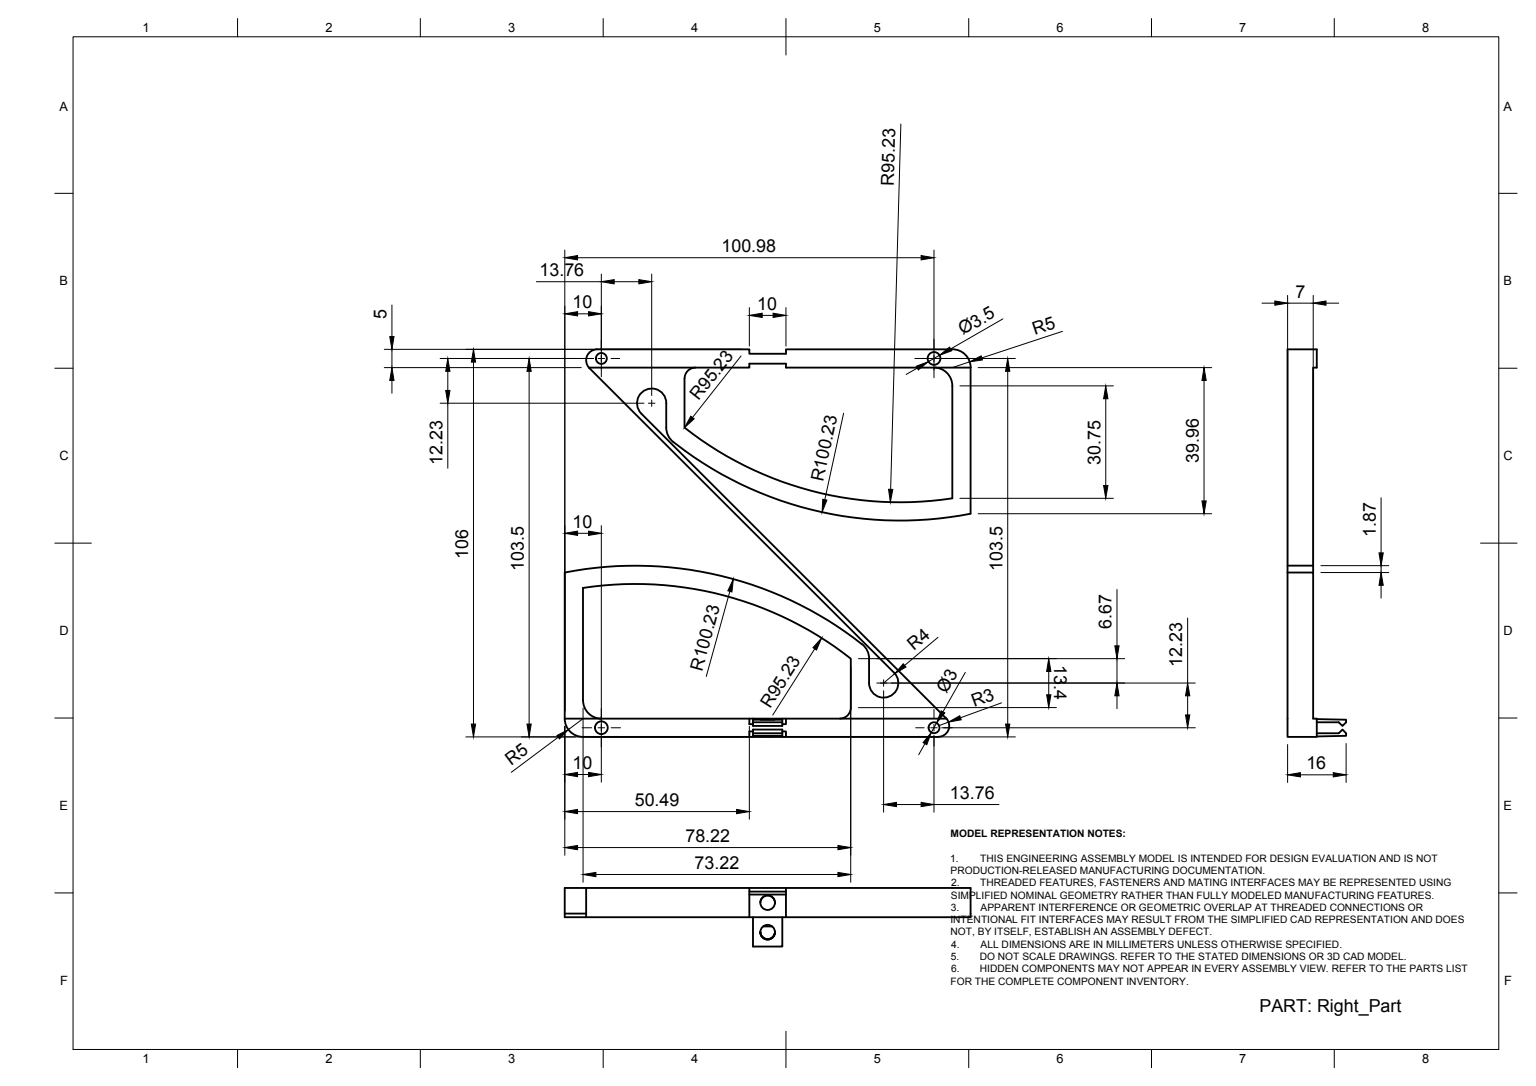
ISO-10303-21;
HEADER;
/* Generated by software containing ST-Developer
 * from STEP Tools, Inc. (www.steptools.com) 
 */

FILE_DESCRIPTION(
/* description */ (''),
/* implementation_level */ '2;1');

FILE_NAME(
/* name */ 'Right_Part.step',
/* time_stamp */ '2026-10-05T13:12:53-07:00',
/* author */ (''),
/* organization */ (''),
/* preprocessor_version */ 'ST-DEVELOPER v20.2',
/* originating_system */ 'Autodesk Translation Framework v15.15.0.0',
/* authorisation */ '');

FILE_SCHEMA (('AUTOMOTIVE_DESIGN { 1 0 10303 214 3 1 1 }'));
ENDSEC;

DATA;
#10=MECHANICAL_DESIGN_GEOMETRIC_PRESENTATION_REPRESENTATION('',(#60),#5912);
#44=SHAPE_REPRESENTATION_RELATIONSHIP('SRR','None',#5945,#52);
#52=ADVANCED_BREP_SHAPE_REPRESENTATION('',(#68),#5905);
#60=STYLED_ITEM('',(#5993),#68);
#68=MANIFOLD_SOLID_BREP('Body1',#3471);
#86=FACE_BOUND('',#473,.T.);
#87=FACE_BOUND('',#474,.T.);
#88=FACE_BOUND('',#485,.T.);
#89=FACE_BOUND('',#489,.T.);
#90=FACE_BOUND('',#510,.T.);
#91=FACE_BOUND('',#511,.T.);
#92=FACE_BOUND('',#513,.T.);
#93=FACE_BOUND('',#515,.T.);
#94=FACE_BOUND('',#516,.T.);
#95=FACE_BOUND('',#522,.T.);
#104=ELLIPSE('',#3708,2.00043399581457,2.);
#105=ELLIPSE('',#3709,2.88922534092348,2.);
#106=ELLIPSE('',#3710,2.00043399581457,2.);
#107=ELLIPSE('',#3711,2.00173692551084,2.);
#108=ELLIPSE('',#3712,2.00173692551084,2.);
#109=ELLIPSE('',#3715,2.00043399581457,2.);
#110=ELLIPSE('',#3716,2.77129645175522,2.);
#111=ELLIPSE('',#3717,2.00043399581457,2.);
#112=ELLIPSE('',#3721,2.00043399581457,2.);
#113=ELLIPSE('',#3722,2.00043399581457,2.);
#138=CYLINDRICAL_SURFACE('',#3707,2.);
#139=CYLINDRICAL_SURFACE('',#3713,2.);
#140=CYLINDRICAL_SURFACE('',#3720,2.);
#141=CYLINDRICAL_SURFACE('',#3723,1.50000013517123);
#142=CYLINDRICAL_SURFACE('',#3727,1.4999996247669);
#143=CYLINDRICAL_SURFACE('',#3732,5.);
#144=CYLINDRICAL_SURFACE('',#3735,5.);
#145=CYLINDRICAL_SURFACE('',#3739,1.75000228959638);
#146=CYLINDRICAL_SURFACE('',#3747,3.00000000000001);
#147=CYLINDRICAL_SURFACE('',#3751,3.99998589024062);
#148=CYLINDRICAL_SURFACE('',#3755,5.00000220964233);
#149=CYLINDRICAL_SURFACE('',#3758,95.231846914414);
#150=CYLINDRICAL_SURFACE('',#3762,3.00000000000008);
#151=CYLINDRICAL_SURFACE('',#3766,2.99999999999999);
#152=CYLINDRICAL_SURFACE('',#3779,100.231846914414);
#153=CYLINDRICAL_SURFACE('',#3794,1.74999969554324);
#154=CYLINDRICAL_SURFACE('',#3798,4.99999999999999);
#155=CYLINDRICAL_SURFACE('',#3801,5.);
#156=CYLINDRICAL_SURFACE('',#3820,100.231846914414);
#157=CYLINDRICAL_SURFACE('',#3832,3.00000000000007);
#158=CYLINDRICAL_SURFACE('',#3834,95.2318469144141);
#159=CYLINDRICAL_SURFACE('',#3836,5.00000220964233);
#160=CYLINDRICAL_SURFACE('',#3838,3.99998589024062);
#161=CYLINDRICAL_SURFACE('',#3840,2.99999999999999);
#250=FACE_OUTER_BOUND('',#443,.T.);
#251=FACE_OUTER_BOUND('',#444,.T.);
#252=FACE_OUTER_BOUND('',#445,.T.);
#253=FACE_OUTER_BOUND('',#446,.T.);
#254=FACE_OUTER_BOUND('',#447,.T.);
#255=FACE_OUTER_BOUND('',#448,.T.);
#256=FACE_OUTER_BOUND('',#449,.T.);
#257=FACE_OUTER_BOUND('',#450,.T.);
#258=FACE_OUTER_BOUND('',#451,.T.);
#259=FACE_OUTER_BOUND('',#452,.T.);
#260=FACE_OUTER_BOUND('',#453,.T.);
#261=FACE_OUTER_BOUND('',#454,.T.);
#262=FACE_OUTER_BOUND('',#455,.T.);
#263=FACE_OUTER_BOUND('',#456,.T.);
#264=FACE_OUTER_BOUND('',#457,.T.);
#265=FACE_OUTER_BOUND('',#458,.T.);
#266=FACE_OUTER_BOUND('',#459,.T.);
#267=FACE_OUTER_BOUND('',#460,.T.);
#268=FACE_OUTER_BOUND('',#461,.T.);
#269=FACE_OUTER_BOUND('',#462,.T.);
#270=FACE_OUTER_BOUND('',#463,.T.);
#271=FACE_OUTER_BOUND('',#464,.T.);
#272=FACE_OUTER_BOUND('',#465,.T.);
#273=FACE_OUTER_BOUND('',#466,.T.);
#274=FACE_OUTER_BOUND('',#467,.T.);
#275=FACE_OUTER_BOUND('',#468,.T.);
#276=FACE_OUTER_BOUND('',#469,.T.);
#277=FACE_OUTER_BOUND('',#470,.T.);
#278=FACE_OUTER_BOUND('',#471,.T.);
#279=FACE_OUTER_BOUND('',#472,.T.);
#280=FACE_OUTER_BOUND('',#475,.T.);
#281=FACE_OUTER_BOUND('',#476,.T.);
#282=FACE_OUTER_BOUND('',#477,.T.);
#283=FACE_OUTER_BOUND('',#478,.T.);
#284=FACE_OUTER_BOUND('',#479,.T.);
#285=FACE_OUTER_BOUND('',#480,.T.);
#286=FACE_OUTER_BOUND('',#481,.T.);
#287=FACE_OUTER_BOUND('',#482,.T.);
#288=FACE_OUTER_BOUND('',#483,.T.);
#289=FACE_OUTER_BOUND('',#484,.T.);
#290=FACE_OUTER_BOUND('',#486,.T.);
#291=FACE_OUTER_BOUND('',#487,.T.);
#292=FACE_OUTER_BOUND('',#488,.T.);
#293=FACE_OUTER_BOUND('',#490,.T.);
#294=FACE_OUTER_BOUND('',#491,.T.);
#295=FACE_OUTER_BOUND('',#492,.T.);
#296=FACE_OUTER_BOUND('',#493,.T.);
#297=FACE_OUTER_BOUND('',#494,.T.);
#298=FACE_OUTER_BOUND('',#495,.T.);
#299=FACE_OUTER_BOUND('',#496,.T.);
#300=FACE_OUTER_BOUND('',#497,.T.);
#301=FACE_OUTER_BOUND('',#498,.T.);
#302=FACE_OUTER_BOUND('',#499,.T.);
#303=FACE_OUTER_BOUND('',#500,.T.);
#304=FACE_OUTER_BOUND('',#501,.T.);
#305=FACE_OUTER_BOUND('',#502,.T.);
#306=FACE_OUTER_BOUND('',#503,.T.);
#307=FACE_OUTER_BOUND('',#504,.T.);
#308=FACE_OUTER_BOUND('',#505,.T.);
#309=FACE_OUTER_BOUND('',#506,.T.);
#310=FACE_OUTER_BOUND('',#507,.T.);
#311=FACE_OUTER_BOUND('',#508,.T.);
#312=FACE_OUTER_BOUND('',#509,.T.);
#313=FACE_OUTER_BOUND('',#512,.T.);
#314=FACE_OUTER_BOUND('',#514,.T.);
#315=FACE_OUTER_BOUND('',#517,.T.);
#316=FACE_OUTER_BOUND('',#518,.T.);
#317=FACE_OUTER_BOUND('',#519,.T.);
#318=FACE_OUTER_BOUND('',#520,.T.);
#319=FACE_OUTER_BOUND('',#521,.T.);
#320=FACE_OUTER_BOUND('',#523,.T.);
#321=FACE_OUTER_BOUND('',#524,.T.);
#322=FACE_OUTER_BOUND('',#525,.T.);
#323=FACE_OUTER_BOUND('',#526,.T.);
#324=FACE_OUTER_BOUND('',#527,.T.);
#325=FACE_OUTER_BOUND('',#528,.T.);
#326=FACE_OUTER_BOUND('',#529,.T.);
#327=FACE_OUTER_BOUND('',#530,.T.);
#328=FACE_OUTER_BOUND('',#531,.T.);
#329=FACE_OUTER_BOUND('',#532,.T.);
#330=FACE_OUTER_BOUND('',#533,.T.);
#331=FACE_OUTER_BOUND('',#534,.T.);
#443=EDGE_LOOP('',(#2654,#2655));
#444=EDGE_LOOP('',(#2656,#2657,#2658,#2659,#2660,#2661,#2662,#2663));
#445=EDGE_LOOP('',(#2664,#2665,#2666,#2667,#2668,#2669));
#446=EDGE_LOOP('',(#2670,#2671,#2672,#2673,#2674,#2675,#2676));
#447=EDGE_LOOP('',(#2677,#2678,#2679,#2680,#2681,#2682,#2683));
#448=EDGE_LOOP('',(#2684,#2685,#2686,#2687));
#449=EDGE_LOOP('',(#2688,#2689,#2690,#2691));
#450=EDGE_LOOP('',(#2692));
#451=EDGE_LOOP('',(#2693,#2694,#2695,#2696));
#452=EDGE_LOOP('',(#2697));
#453=EDGE_LOOP('',(#2698,#2699,#2700,#2701));
#454=EDGE_LOOP('',(#2702,#2703,#2704,#2705,#2706));
#455=EDGE_LOOP('',(#2707,#2708,#2709,#2710));
#456=EDGE_LOOP('',(#2711,#2712,#2713,#2714));
#457=EDGE_LOOP('',(#2715,#2716,#2717,#2718));
#458=EDGE_LOOP('',(#2719));
#459=EDGE_LOOP('',(#2720,#2721,#2722,#2723));
#460=EDGE_LOOP('',(#2724,#2725,#2726,#2727));
#461=EDGE_LOOP('',(#2728,#2729,#2730,#2731,#2732,#2733));
#462=EDGE_LOOP('',(#2734,#2735,#2736,#2737,#2738,#2739));
#463=EDGE_LOOP('',(#2740,#2741,#2742,#2743,#2744));
#464=EDGE_LOOP('',(#2745,#2746,#2747,#2748));
#465=EDGE_LOOP('',(#2749,#2750,#2751,#2752));
#466=EDGE_LOOP('',(#2753,#2754,#2755,#2756));
#467=EDGE_LOOP('',(#2757,#2758,#2759,#2760));
#468=EDGE_LOOP('',(#2761,#2762,#2763,#2764));
#469=EDGE_LOOP('',(#2765,#2766,#2767,#2768));
#470=EDGE_LOOP('',(#2769,#2770,#2771,#2772,#2773,#2774,#2775,#2776,#2777,
#2778,#2779,#2780,#2781,#2782));
#471=EDGE_LOOP('',(#2783,#2784,#2785,#2786));
#472=EDGE_LOOP('',(#2787,#2788,#2789,#2790,#2791,#2792,#2793,#2794,#2795,
#2796,#2797,#2798));
#473=EDGE_LOOP('',(#2799));
#474=EDGE_LOOP('',(#2800));
#475=EDGE_LOOP('',(#2801,#2802,#2803,#2804));
#476=EDGE_LOOP('',(#2805,#2806,#2807,#2808));
#477=EDGE_LOOP('',(#2809,#2810,#2811,#2812));
#478=EDGE_LOOP('',(#2813,#2814,#2815,#2816,#2817,#2818));
#479=EDGE_LOOP('',(#2819,#2820,#2821,#2822,#2823,#2824,#2825,#2826));
#480=EDGE_LOOP('',(#2827,#2828,#2829,#2830,#2831,#2832));
#481=EDGE_LOOP('',(#2833,#2834,#2835,#2836));
#482=EDGE_LOOP('',(#2837,#2838,#2839,#2840));
#483=EDGE_LOOP('',(#2841,#2842,#2843,#2844,#2845,#2846));
#484=EDGE_LOOP('',(#2847,#2848,#2849,#2850));
#485=EDGE_LOOP('',(#2851));
#486=EDGE_LOOP('',(#2852,#2853,#2854,#2855));
#487=EDGE_LOOP('',(#2856,#2857,#2858,#2859,#2860,#2861,#2862,#2863,#2864,
#2865,#2866));
#488=EDGE_LOOP('',(#2867,#2868,#2869,#2870));
#489=EDGE_LOOP('',(#2871,#2872,#2873));
#490=EDGE_LOOP('',(#2874,#2875,#2876,#2877));
#491=EDGE_LOOP('',(#2878,#2879,#2880,#2881));
#492=EDGE_LOOP('',(#2882,#2883,#2884,#2885,#2886,#2887));
#493=EDGE_LOOP('',(#2888,#2889,#2890,#2891,#2892,#2893,#2894,#2895));
#494=EDGE_LOOP('',(#2896,#2897,#2898,#2899));
#495=EDGE_LOOP('',(#2900,#2901,#2902,#2903,#2904,#2905));
#496=EDGE_LOOP('',(#2906,#2907,#2908,#2909,#2910,#2911));
#497=EDGE_LOOP('',(#2912,#2913,#2914,#2915,#2916));
#498=EDGE_LOOP('',(#2917));
#499=EDGE_LOOP('',(#2918,#2919,#2920,#2921));
#500=EDGE_LOOP('',(#2922,#2923,#2924,#2925,#2926,#2927));
#501=EDGE_LOOP('',(#2928,#2929,#2930,#2931));
#502=EDGE_LOOP('',(#2932,#2933,#2934,#2935));
#503=EDGE_LOOP('',(#2936,#2937,#2938,#2939,#2940,#2941));
#504=EDGE_LOOP('',(#2942,#2943,#2944,#2945));
#505=EDGE_LOOP('',(#2946,#2947,#2948,#2949));
#506=EDGE_LOOP('',(#2950,#2951,#2952,#2953));
#507=EDGE_LOOP('',(#2954,#2955,#2956,#2957));
#508=EDGE_LOOP('',(#2958,#2959,#2960,#2961));
#509=EDGE_LOOP('',(#2962,#2963,#2964,#2965,#2966,#2967,#2968,#2969,#2970,
#2971,#2972,#2973,#2974,#2975,#2976,#2977,#2978,#2979,#2980,#2981,#2982,
#2983,#2984));
#510=EDGE_LOOP('',(#2985,#2986,#2987,#2988,#2989,#2990,#2991,#2992,#2993,
#2994));
#511=EDGE_LOOP('',(#2995,#2996,#2997,#2998,#2999,#3000));
#512=EDGE_LOOP('',(#3001,#3002,#3003,#3004));
#513=EDGE_LOOP('',(#3005));
#514=EDGE_LOOP('',(#3006,#3007,#3008,#3009,#3010,#3011,#3012,#3013,#3014,
#3015,#3016,#3017));
#515=EDGE_LOOP('',(#3018));
#516=EDGE_LOOP('',(#3019));
#517=EDGE_LOOP('',(#3020,#3021,#3022,#3023));
#518=EDGE_LOOP('',(#3024,#3025,#3026,#3027));
#519=EDGE_LOOP('',(#3028,#3029,#3030,#3031,#3032,#3033,#3034,#3035,#3036,
#3037,#3038,#3039,#3040,#3041,#3042,#3043,#3044,#3045,#3046,#3047,#3048,
#3049,#3050,#3051,#3052,#3053,#3054,#3055,#3056));
#520=EDGE_LOOP('',(#3057,#3058,#3059,#3060,#3061,#3062));
#521=EDGE_LOOP('',(#3063,#3064,#3065,#3066));
#522=EDGE_LOOP('',(#3067));
#523=EDGE_LOOP('',(#3068,#3069,#3070,#3071,#3072,#3073));
#524=EDGE_LOOP('',(#3074,#3075,#3076,#3077,#3078,#3079));
#525=EDGE_LOOP('',(#3080,#3081,#3082,#3083));
#526=EDGE_LOOP('',(#3084,#3085,#3086,#3087));
#527=EDGE_LOOP('',(#3088,#3089,#3090,#3091));
#528=EDGE_LOOP('',(#3092,#3093,#3094,#3095));
#529=EDGE_LOOP('',(#3096,#3097,#3098,#3099));
#530=EDGE_LOOP('',(#3100,#3101,#3102,#3103));
#531=EDGE_LOOP('',(#3104,#3105,#3106,#3107));
#532=EDGE_LOOP('',(#3108,#3109,#3110,#3111,#3112));
#533=EDGE_LOOP('',(#3113,#3114,#3115,#3116,#3117,#3118,#3119));
#534=EDGE_LOOP('',(#3120,#3121,#3122,#3123));
#598=CIRCLE('',#3706,2.);
#599=CIRCLE('',#3714,2.);
#600=CIRCLE('',#3724,1.50000013517123);
#601=CIRCLE('',#3725,1.50000013517123);
#602=CIRCLE('',#3728,1.4999996247669);
#603=CIRCLE('',#3729,1.4999996247669);
#604=CIRCLE('',#3733,5.);
#605=CIRCLE('',#3734,5.);
#606=CIRCLE('',#3736,5.);
#607=CIRCLE('',#3737,5.);
#608=CIRCLE('',#3740,1.75000228959638);
#609=CIRCLE('',#3741,1.75000228959638);
#610=CIRCLE('',#3748,3.00000000000001);
#611=CIRCLE('',#3749,3.00000000000001);
#612=CIRCLE('',#3750,3.00000000000001);
#613=CIRCLE('',#3752,3.99998589024062);
#614=CIRCLE('',#3753,3.99998589024062);
#615=CIRCLE('',#3756,5.00000220964233);
#616=CIRCLE('',#3757,5.00000220964233);
#617=CIRCLE('',#3759,95.231846914414);
#618=CIRCLE('',#3760,95.231846914414);
#619=CIRCLE('',#3763,3.00000000000008);
#620=CIRCLE('',#3764,3.00000000000008);
#621=CIRCLE('',#3767,2.99999999999999);
#622=CIRCLE('',#3780,100.231846914414);
#623=CIRCLE('',#3781,100.231846914414);
#624=CIRCLE('',#3793,1.74999969554324);
#625=CIRCLE('',#3795,1.74999969554324);
#626=CIRCLE('',#3799,4.99999999999999);
#627=CIRCLE('',#3800,4.99999999999999);
#628=CIRCLE('',#3802,5.);
#629=CIRCLE('',#3803,5.);
#630=CIRCLE('',#3810,2.99999999999999);
#631=CIRCLE('',#3811,100.231846914414);
#632=CIRCLE('',#3812,5.00000220964233);
#633=CIRCLE('',#3813,3.99998589024062);
#634=CIRCLE('',#3814,3.00000000000007);
#635=CIRCLE('',#3815,95.2318469144141);
#636=CIRCLE('',#3818,2.99999999999999);
#637=CIRCLE('',#3821,100.231846914414);
#638=CIRCLE('',#3823,3.99998589024062);
#639=CIRCLE('',#3824,5.00000220964233);
#640=CIRCLE('',#3825,95.2318469144141);
#641=CIRCLE('',#3826,3.00000000000007);
#642=CIRCLE('',#3827,2.99999999999999);
#834=LINE('',#5362,#1199);
#835=LINE('',#5372,#1200);
#836=LINE('',#5379,#1201);
#837=LINE('',#5387,#1202);
#838=LINE('',#5389,#1203);
#839=LINE('',#5391,#1204);
#840=LINE('',#5393,#1205);
#841=LINE('',#5394,#1206);
#842=LINE('',#5397,#1207);
#843=LINE('',#5399,#1208);
#844=LINE('',#5401,#1209);
#845=LINE('',#5403,#1210);
#846=LINE('',#5404,#1211);
#847=LINE('',#5409,#1212);
#848=LINE('',#5415,#1213);
#849=LINE('',#5422,#1214);
#850=LINE('',#5428,#1215);
#851=LINE('',#5430,#1216);
#852=LINE('',#5432,#1217);
#853=LINE('',#5433,#1218);
#854=LINE('',#5438,#1219);
#855=LINE('',#5441,#1220);
#856=LINE('',#5447,#1221);
#857=LINE('',#5450,#1222);
#858=LINE('',#5453,#1223);
#859=LINE('',#5455,#1224);
#860=LINE('',#5456,#1225);
#861=LINE('',#5461,#1226);
#862=LINE('',#5467,#1227);
#863=LINE('',#5469,#1228);
#864=LINE('',#5471,#1229);
#865=LINE('',#5472,#1230);
#866=LINE('',#5476,#1231);
#867=LINE('',#5478,#1232);
#868=LINE('',#5480,#1233);
#869=LINE('',#5481,#1234);
#870=LINE('',#5485,#1235);
#871=LINE('',#5487,#1236);
#872=LINE('',#5488,#1237);
#873=LINE('',#5490,#1238);
#874=LINE('',#5491,#1239);
#875=LINE('',#5495,#1240);
#876=LINE('',#5497,#1241);
#877=LINE('',#5498,#1242);
#878=LINE('',#5500,#1243);
#879=LINE('',#5501,#1244);
#880=LINE('',#5507,#1245);
#881=LINE('',#5512,#1246);
#882=LINE('',#5518,#1247);
#883=LINE('',#5521,#1248);
#884=LINE('',#5524,#1249);
#885=LINE('',#5526,#1250);
#886=LINE('',#5527,#1251);
#887=LINE('',#5532,#1252);
#888=LINE('',#5538,#1253);
#889=LINE('',#5542,#1254);
#890=LINE('',#5544,#1255);
#891=LINE('',#5545,#1256);
#892=LINE('',#5550,#1257);
#893=LINE('',#5554,#1258);
#894=LINE('',#5556,#1259);
#895=LINE('',#5558,#1260);
#896=LINE('',#5560,#1261);
#897=LINE('',#5561,#1262);
#898=LINE('',#5562,#1263);
#899=LINE('',#5563,#1264);
#900=LINE('',#5564,#1265);
#901=LINE('',#5565,#1266);
#902=LINE('',#5566,#1267);
#903=LINE('',#5570,#1268);
#904=LINE('',#5573,#1269);
#905=LINE('',#5575,#1270);
#906=LINE('',#5576,#1271);
#907=LINE('',#5578,#1272);
#908=LINE('',#5579,#1273);
#909=LINE('',#5580,#1274);
#910=LINE('',#5583,#1275);
#911=LINE('',#5584,#1276);
#912=LINE('',#5586,#1277);
#913=LINE('',#5589,#1278);
#914=LINE('',#5591,#1279);
#915=LINE('',#5592,#1280);
#916=LINE('',#5596,#1281);
#917=LINE('',#5598,#1282);
#918=LINE('',#5599,#1283);
#919=LINE('',#5601,#1284);
#920=LINE('',#5602,#1285);
#921=LINE('',#5604,#1286);
#922=LINE('',#5608,#1287);
#923=LINE('',#5610,#1288);
#924=LINE('',#5611,#1289);
#925=LINE('',#5612,#1290);
#926=LINE('',#5614,#1291);
#927=LINE('',#5615,#1292);
#928=LINE('',#5617,#1293);
#929=LINE('',#5624,#1294);
#930=LINE('',#5625,#1295);
#931=LINE('',#5626,#1296);
#932=LINE('',#5627,#1297);
#933=LINE('',#5629,#1298);
#934=LINE('',#5631,#1299);
#935=LINE('',#5633,#1300);
#936=LINE('',#5636,#1301);
#937=LINE('',#5641,#1302);
#938=LINE('',#5643,#1303);
#939=LINE('',#5645,#1304);
#940=LINE('',#5647,#1305);
#941=LINE('',#5649,#1306);
#942=LINE('',#5650,#1307);
#943=LINE('',#5654,#1308);
#944=LINE('',#5656,#1309);
#945=LINE('',#5658,#1310);
#946=LINE('',#5660,#1311);
#947=LINE('',#5662,#1312);
#948=LINE('',#5663,#1313);
#949=LINE('',#5666,#1314);
#950=LINE('',#5668,#1315);
#951=LINE('',#5670,#1316);
#952=LINE('',#5671,#1317);
#953=LINE('',#5677,#1318);
#954=LINE('',#5681,#1319);
#955=LINE('',#5683,#1320);
#956=LINE('',#5685,#1321);
#957=LINE('',#5687,#1322);
#958=LINE('',#5688,#1323);
#959=LINE('',#5692,#1324);
#960=LINE('',#5694,#1325);
#961=LINE('',#5696,#1326);
#962=LINE('',#5697,#1327);
#963=LINE('',#5705,#1328);
#964=LINE('',#5708,#1329);
#965=LINE('',#5710,#1330);
#966=LINE('',#5711,#1331);
#967=LINE('',#5714,#1332);
#968=LINE('',#5716,#1333);
#969=LINE('',#5717,#1334);
#970=LINE('',#5720,#1335);
#971=LINE('',#5721,#1336);
#972=LINE('',#5724,#1337);
#973=LINE('',#5726,#1338);
#974=LINE('',#5727,#1339);
#975=LINE('',#5730,#1340);
#976=LINE('',#5731,#1341);
#977=LINE('',#5734,#1342);
#978=LINE('',#5738,#1343);
#979=LINE('',#5739,#1344);
#980=LINE('',#5743,#1345);
#981=LINE('',#5747,#1346);
#982=LINE('',#5750,#1347);
#983=LINE('',#5752,#1348);
#984=LINE('',#5754,#1349);
#985=LINE('',#5758,#1350);
#986=LINE('',#5762,#1351);
#987=LINE('',#5763,#1352);
#988=LINE('',#5766,#1353);
#989=LINE('',#5768,#1354);
#990=LINE('',#5770,#1355);
#991=LINE('',#5774,#1356);
#992=LINE('',#5775,#1357);
#993=LINE('',#5778,#1358);
#994=LINE('',#5779,#1359);
#995=LINE('',#5783,#1360);
#996=LINE('',#5786,#1361);
#997=LINE('',#5790,#1362);
#998=LINE('',#5793,#1363);
#999=LINE('',#5797,#1364);
#1000=LINE('',#5801,#1365);
#1001=LINE('',#5804,#1366);
#1002=LINE('',#5806,#1367);
#1003=LINE('',#5808,#1368);
#1004=LINE('',#5810,#1369);
#1005=LINE('',#5811,#1370);
#1006=LINE('',#5813,#1371);
#1007=LINE('',#5815,#1372);
#1008=LINE('',#5818,#1373);
#1009=LINE('',#5820,#1374);
#1010=LINE('',#5822,#1375);
#1011=LINE('',#5824,#1376);
#1012=LINE('',#5827,#1377);
#1013=LINE('',#5828,#1378);
#1199=VECTOR('',#4343,10.);
#1200=VECTOR('',#4354,2.);
#1201=VECTOR('',#4363,2.);
#1202=VECTOR('',#4372,10.);
#1203=VECTOR('',#4373,10.);
#1204=VECTOR('',#4374,10.);
#1205=VECTOR('',#4375,10.);
#1206=VECTOR('',#4376,10.);
#1207=VECTOR('',#4379,10.);
#1208=VECTOR('',#4380,10.);
#1209=VECTOR('',#4381,10.);
#1210=VECTOR('',#4382,10.);
#1211=VECTOR('',#4383,10.);
#1212=VECTOR('',#4388,2.);
#1213=VECTOR('',#4395,1.50000013517123);
#1214=VECTOR('',#4404,1.4999996247669);
#1215=VECTOR('',#4411,10.);
#1216=VECTOR('',#4412,10.);
#1217=VECTOR('',#4413,10.);
#1218=VECTOR('',#4414,10.);
#1219=VECTOR('',#4419,10.);
#1220=VECTOR('',#4422,10.);
#1221=VECTOR('',#4427,10.);
#1222=VECTOR('',#4430,10.);
#1223=VECTOR('',#4433,10.);
#1224=VECTOR('',#4434,10.);
#1225=VECTOR('',#4435,10.);
#1226=VECTOR('',#4440,1.75000228959638);
#1227=VECTOR('',#4447,10.);
#1228=VECTOR('',#4448,10.);
#1229=VECTOR('',#4449,10.);
#1230=VECTOR('',#4450,10.);
#1231=VECTOR('',#4453,10.);
#1232=VECTOR('',#4454,10.);
#1233=VECTOR('',#4455,10.);
#1234=VECTOR('',#4456,10.);
#1235=VECTOR('',#4459,10.);
#1236=VECTOR('',#4460,10.);
#1237=VECTOR('',#4461,10.);
#1238=VECTOR('',#4462,10.);
#1239=VECTOR('',#4463,10.);
#1240=VECTOR('',#4466,10.);
#1241=VECTOR('',#4467,10.);
#1242=VECTOR('',#4468,10.);
#1243=VECTOR('',#4469,10.);
#1244=VECTOR('',#4470,10.);
#1245=VECTOR('',#4475,10.);
#1246=VECTOR('',#4480,10.);
#1247=VECTOR('',#4485,10.);
#1248=VECTOR('',#4488,10.);
#1249=VECTOR('',#4491,10.);
#1250=VECTOR('',#4492,10.);
#1251=VECTOR('',#4493,10.);
#1252=VECTOR('',#4498,10.);
#1253=VECTOR('',#4505,10.);
#1254=VECTOR('',#4510,9.99999999999999);
#1255=VECTOR('',#4511,10.);
#1256=VECTOR('',#4512,9.99999999999999);
#1257=VECTOR('',#4517,10.);
#1258=VECTOR('',#4522,10.);
#1259=VECTOR('',#4523,10.);
#1260=VECTOR('',#4524,10.);
#1261=VECTOR('',#4525,10.);
#1262=VECTOR('',#4526,10.);
#1263=VECTOR('',#4527,10.);
#1264=VECTOR('',#4528,10.);
#1265=VECTOR('',#4529,10.);
#1266=VECTOR('',#4530,10.);
#1267=VECTOR('',#4531,10.);
#1268=VECTOR('',#4536,10.);
#1269=VECTOR('',#4539,10.);
#1270=VECTOR('',#4540,10.);
#1271=VECTOR('',#4541,10.);
#1272=VECTOR('',#4542,10.);
#1273=VECTOR('',#4543,10.);
#1274=VECTOR('',#4544,10.);
#1275=VECTOR('',#4547,10.);
#1276=VECTOR('',#4548,10.);
#1277=VECTOR('',#4551,10.);
#1278=VECTOR('',#4554,10.);
#1279=VECTOR('',#4555,10.);
#1280=VECTOR('',#4556,10.);
#1281=VECTOR('',#4559,10.);
#1282=VECTOR('',#4560,10.);
#1283=VECTOR('',#4561,10.);
#1284=VECTOR('',#4562,10.);
#1285=VECTOR('',#4563,10.);
#1286=VECTOR('',#4566,10.);
#1287=VECTOR('',#4569,10.);
#1288=VECTOR('',#4570,10.);
#1289=VECTOR('',#4571,10.);
#1290=VECTOR('',#4572,10.);
#1291=VECTOR('',#4575,10.);
#1292=VECTOR('',#4576,10.);
#1293=VECTOR('',#4579,10.);
#1294=VECTOR('',#4592,10.);
#1295=VECTOR('',#4593,10.);
#1296=VECTOR('',#4594,10.);
#1297=VECTOR('',#4595,10.);
#1298=VECTOR('',#4598,10.);
#1299=VECTOR('',#4601,10.);
#1300=VECTOR('',#4604,10.);
#1301=VECTOR('',#4609,10.);
#1302=VECTOR('',#4614,10.);
#1303=VECTOR('',#4615,10.);
#1304=VECTOR('',#4616,10.);
#1305=VECTOR('',#4617,10.);
#1306=VECTOR('',#4618,10.);
#1307=VECTOR('',#4619,10.);
#1308=VECTOR('',#4622,10.);
#1309=VECTOR('',#4623,10.);
#1310=VECTOR('',#4624,10.);
#1311=VECTOR('',#4625,10.);
#1312=VECTOR('',#4626,10.);
#1313=VECTOR('',#4627,10.);
#1314=VECTOR('',#4630,10.);
#1315=VECTOR('',#4631,10.);
#1316=VECTOR('',#4632,10.);
#1317=VECTOR('',#4633,10.);
#1318=VECTOR('',#4640,1.74999969554324);
#1319=VECTOR('',#4645,10.);
#1320=VECTOR('',#4646,10.);
#1321=VECTOR('',#4647,10.);
#1322=VECTOR('',#4648,10.);
#1323=VECTOR('',#4649,10.);
#1324=VECTOR('',#4652,10.);
#1325=VECTOR('',#4653,10.);
#1326=VECTOR('',#4654,10.);
#1327=VECTOR('',#4655,10.);
#1328=VECTOR('',#4668,10.);
#1329=VECTOR('',#4671,10.);
#1330=VECTOR('',#4672,10.);
#1331=VECTOR('',#4673,10.);
#1332=VECTOR('',#4676,10.);
#1333=VECTOR('',#4677,10.);
#1334=VECTOR('',#4678,10.);
#1335=VECTOR('',#4681,10.);
#1336=VECTOR('',#4682,10.);
#1337=VECTOR('',#4685,10.);
#1338=VECTOR('',#4686,10.);
#1339=VECTOR('',#4687,10.);
#1340=VECTOR('',#4690,10.);
#1341=VECTOR('',#4691,10.);
#1342=VECTOR('',#4694,10.);
#1343=VECTOR('',#4697,10.);
#1344=VECTOR('',#4698,10.);
#1345=VECTOR('',#4701,10.);
#1346=VECTOR('',#4704,10.);
#1347=VECTOR('',#4707,10.);
#1348=VECTOR('',#4708,10.);
#1349=VECTOR('',#4709,10.);
#1350=VECTOR('',#4712,9.99999999999999);
#1351=VECTOR('',#4717,10.);
#1352=VECTOR('',#4718,10.);
#1353=VECTOR('',#4721,10.);
#1354=VECTOR('',#4722,10.);
#1355=VECTOR('',#4723,10.);
#1356=VECTOR('',#4726,10.);
#1357=VECTOR('',#4727,10.);
#1358=VECTOR('',#4730,10.);
#1359=VECTOR('',#4731,10.);
#1360=VECTOR('',#4736,10.);
#1361=VECTOR('',#4739,10.);
#1362=VECTOR('',#4742,10.);
#1363=VECTOR('',#4745,10.);
#1364=VECTOR('',#4748,9.99999999999999);
#1365=VECTOR('',#4751,10.);
#1366=VECTOR('',#4756,10.);
#1367=VECTOR('',#4759,10.);
#1368=VECTOR('',#4762,10.);
#1369=VECTOR('',#4765,10.);
#1370=VECTOR('',#4766,10.);
#1371=VECTOR('',#4769,10.);
#1372=VECTOR('',#4772,10.);
#1373=VECTOR('',#4777,10.);
#1374=VECTOR('',#4780,10.);
#1375=VECTOR('',#4783,10.);
#1376=VECTOR('',#4786,10.);
#1377=VECTOR('',#4789,10.);
#1378=VECTOR('',#4790,10.);
#1538=VERTEX_POINT('',#5360);
#1539=VERTEX_POINT('',#5361);
#1540=VERTEX_POINT('',#5365);
#1541=VERTEX_POINT('',#5366);
#1542=VERTEX_POINT('',#5368);
#1543=VERTEX_POINT('',#5371);
#1544=VERTEX_POINT('',#5376);
#1545=VERTEX_POINT('',#5378);
#1546=VERTEX_POINT('',#5380);
#1547=VERTEX_POINT('',#5382);
#1548=VERTEX_POINT('',#5386);
#1549=VERTEX_POINT('',#5388);
#1550=VERTEX_POINT('',#5390);
#1551=VERTEX_POINT('',#5392);
#1552=VERTEX_POINT('',#5396);
#1553=VERTEX_POINT('',#5398);
#1554=VERTEX_POINT('',#5400);
#1555=VERTEX_POINT('',#5402);
#1556=VERTEX_POINT('',#5406);
#1557=VERTEX_POINT('',#5408);
#1558=VERTEX_POINT('',#5412);
#1559=VERTEX_POINT('',#5414);
#1560=VERTEX_POINT('',#5419);
#1561=VERTEX_POINT('',#5421);
#1562=VERTEX_POINT('',#5426);
#1563=VERTEX_POINT('',#5427);
#1564=VERTEX_POINT('',#5429);
#1565=VERTEX_POINT('',#5431);
#1566=VERTEX_POINT('',#5435);
#1567=VERTEX_POINT('',#5437);
#1568=VERTEX_POINT('',#5439);
#1569=VERTEX_POINT('',#5443);
#1570=VERTEX_POINT('',#5444);
#1571=VERTEX_POINT('',#5446);
#1572=VERTEX_POINT('',#5448);
#1573=VERTEX_POINT('',#5452);
#1574=VERTEX_POINT('',#5454);
#1575=VERTEX_POINT('',#5458);
#1576=VERTEX_POINT('',#5460);
#1577=VERTEX_POINT('',#5465);
#1578=VERTEX_POINT('',#5466);
#1579=VERTEX_POINT('',#5468);
#1580=VERTEX_POINT('',#5470);
#1581=VERTEX_POINT('',#5474);
#1582=VERTEX_POINT('',#5475);
#1583=VERTEX_POINT('',#5477);
#1584=VERTEX_POINT('',#5479);
#1585=VERTEX_POINT('',#5483);
#1586=VERTEX_POINT('',#5484);
#1587=VERTEX_POINT('',#5486);
#1588=VERTEX_POINT('',#5489);
#1589=VERTEX_POINT('',#5493);
#1590=VERTEX_POINT('',#5494);
#1591=VERTEX_POINT('',#5496);
#1592=VERTEX_POINT('',#5499);
#1593=VERTEX_POINT('',#5503);
#1594=VERTEX_POINT('',#5504);
#1595=VERTEX_POINT('',#5506);
#1596=VERTEX_POINT('',#5508);
#1597=VERTEX_POINT('',#5510);
#1598=VERTEX_POINT('',#5514);
#1599=VERTEX_POINT('',#5515);
#1600=VERTEX_POINT('',#5517);
#1601=VERTEX_POINT('',#5519);
#1602=VERTEX_POINT('',#5523);
#1603=VERTEX_POINT('',#5525);
#1604=VERTEX_POINT('',#5529);
#1605=VERTEX_POINT('',#5531);
#1606=VERTEX_POINT('',#5535);
#1607=VERTEX_POINT('',#5537);
#1608=VERTEX_POINT('',#5541);
#1609=VERTEX_POINT('',#5543);
#1610=VERTEX_POINT('',#5547);
#1611=VERTEX_POINT('',#5549);
#1612=VERTEX_POINT('',#5553);
#1613=VERTEX_POINT('',#5555);
#1614=VERTEX_POINT('',#5557);
#1615=VERTEX_POINT('',#5559);
#1616=VERTEX_POINT('',#5568);
#1617=VERTEX_POINT('',#5572);
#1618=VERTEX_POINT('',#5574);
#1619=VERTEX_POINT('',#5577);
#1620=VERTEX_POINT('',#5582);
#1621=VERTEX_POINT('',#5588);
#1622=VERTEX_POINT('',#5590);
#1623=VERTEX_POINT('',#5594);
#1624=VERTEX_POINT('',#5595);
#1625=VERTEX_POINT('',#5597);
#1626=VERTEX_POINT('',#5600);
#1627=VERTEX_POINT('',#5606);
#1628=VERTEX_POINT('',#5607);
#1629=VERTEX_POINT('',#5609);
#1630=VERTEX_POINT('',#5639);
#1631=VERTEX_POINT('',#5640);
#1632=VERTEX_POINT('',#5642);
#1633=VERTEX_POINT('',#5644);
#1634=VERTEX_POINT('',#5646);
#1635=VERTEX_POINT('',#5648);
#1636=VERTEX_POINT('',#5652);
#1637=VERTEX_POINT('',#5653);
#1638=VERTEX_POINT('',#5655);
#1639=VERTEX_POINT('',#5657);
#1640=VERTEX_POINT('',#5659);
#1641=VERTEX_POINT('',#5661);
#1642=VERTEX_POINT('',#5665);
#1643=VERTEX_POINT('',#5667);
#1644=VERTEX_POINT('',#5669);
#1645=VERTEX_POINT('',#5673);
#1646=VERTEX_POINT('',#5676);
#1647=VERTEX_POINT('',#5680);
#1648=VERTEX_POINT('',#5682);
#1649=VERTEX_POINT('',#5684);
#1650=VERTEX_POINT('',#5686);
#1651=VERTEX_POINT('',#5690);
#1652=VERTEX_POINT('',#5691);
#1653=VERTEX_POINT('',#5693);
#1654=VERTEX_POINT('',#5695);
#1655=VERTEX_POINT('',#5702);
#1656=VERTEX_POINT('',#5707);
#1657=VERTEX_POINT('',#5709);
#1658=VERTEX_POINT('',#5713);
#1659=VERTEX_POINT('',#5715);
#1660=VERTEX_POINT('',#5719);
#1661=VERTEX_POINT('',#5723);
#1662=VERTEX_POINT('',#5725);
#1663=VERTEX_POINT('',#5729);
#1664=VERTEX_POINT('',#5733);
#1665=VERTEX_POINT('',#5735);
#1666=VERTEX_POINT('',#5737);
#1667=VERTEX_POINT('',#5740);
#1668=VERTEX_POINT('',#5742);
#1669=VERTEX_POINT('',#5744);
#1670=VERTEX_POINT('',#5746);
#1671=VERTEX_POINT('',#5748);
#1672=VERTEX_POINT('',#5751);
#1673=VERTEX_POINT('',#5753);
#1674=VERTEX_POINT('',#5755);
#1675=VERTEX_POINT('',#5757);
#1676=VERTEX_POINT('',#5761);
#1677=VERTEX_POINT('',#5765);
#1678=VERTEX_POINT('',#5767);
#1679=VERTEX_POINT('',#5769);
#1680=VERTEX_POINT('',#5771);
#1681=VERTEX_POINT('',#5773);
#1682=VERTEX_POINT('',#5777);
#1683=VERTEX_POINT('',#5781);
#1684=VERTEX_POINT('',#5785);
#1685=VERTEX_POINT('',#5787);
#1686=VERTEX_POINT('',#5789);
#1687=VERTEX_POINT('',#5791);
#1688=VERTEX_POINT('',#5794);
#1689=VERTEX_POINT('',#5796);
#1690=VERTEX_POINT('',#5798);
#1691=VERTEX_POINT('',#5800);
#1692=VERTEX_POINT('',#5826);
#1937=EDGE_CURVE('',#1538,#1539,#834,.T.);
#1938=EDGE_CURVE('',#1538,#1539,#598,.T.);
#1939=EDGE_CURVE('',#1540,#1541,#104,.T.);
#1940=EDGE_CURVE('',#1542,#1540,#105,.T.);
#1941=EDGE_CURVE('',#1541,#1542,#106,.T.);
#1942=EDGE_CURVE('',#1541,#1543,#835,.T.);
#1943=EDGE_CURVE('',#1539,#1543,#107,.T.);
#1944=EDGE_CURVE('',#1543,#1538,#108,.T.);
#1945=EDGE_CURVE('',#1544,#1544,#599,.T.);
#1946=EDGE_CURVE('',#1544,#1545,#836,.T.);
#1947=EDGE_CURVE('',#1546,#1545,#109,.T.);
#1948=EDGE_CURVE('',#1547,#1546,#110,.T.);
#1949=EDGE_CURVE('',#1545,#1547,#111,.T.);
#1950=EDGE_CURVE('',#1548,#1547,#837,.T.);
#1951=EDGE_CURVE('',#1549,#1548,#838,.T.);
#1952=EDGE_CURVE('',#1550,#1549,#839,.T.);
#1953=EDGE_CURVE('',#1551,#1550,#840,.T.);
#1954=EDGE_CURVE('',#1546,#1551,#841,.T.);
#1955=EDGE_CURVE('',#1542,#1552,#842,.T.);
#1956=EDGE_CURVE('',#1553,#1552,#843,.T.);
#1957=EDGE_CURVE('',#1554,#1553,#844,.T.);
#1958=EDGE_CURVE('',#1555,#1554,#845,.T.);
#1959=EDGE_CURVE('',#1555,#1540,#846,.T.);
#1960=EDGE_CURVE('',#1556,#1556,#112,.T.);
#1961=EDGE_CURVE('',#1556,#1557,#847,.T.);
#1962=EDGE_CURVE('',#1557,#1557,#113,.T.);
#1963=EDGE_CURVE('',#1558,#1558,#600,.T.);
#1964=EDGE_CURVE('',#1558,#1559,#848,.T.);
#1965=EDGE_CURVE('',#1559,#1559,#601,.T.);
#1966=EDGE_CURVE('',#1560,#1560,#602,.T.);
#1967=EDGE_CURVE('',#1560,#1561,#849,.T.);
#1968=EDGE_CURVE('',#1561,#1561,#603,.T.);
#1969=EDGE_CURVE('',#1562,#1563,#850,.T.);
#1970=EDGE_CURVE('',#1562,#1564,#851,.T.);
#1971=EDGE_CURVE('',#1565,#1564,#852,.T.);
#1972=EDGE_CURVE('',#1563,#1565,#853,.T.);
#1973=EDGE_CURVE('',#1566,#1562,#604,.T.);
#1974=EDGE_CURVE('',#1566,#1567,#854,.T.);
#1975=EDGE_CURVE('',#1568,#1567,#605,.T.);
#1976=EDGE_CURVE('',#1564,#1568,#855,.T.);
#1977=EDGE_CURVE('',#1569,#1570,#606,.T.);
#1978=EDGE_CURVE('',#1569,#1571,#856,.T.);
#1979=EDGE_CURVE('',#1572,#1571,#607,.T.);
#1980=EDGE_CURVE('',#1570,#1572,#857,.T.);
#1981=EDGE_CURVE('',#1573,#1569,#858,.T.);
#1982=EDGE_CURVE('',#1573,#1574,#859,.T.);
#1983=EDGE_CURVE('',#1571,#1574,#860,.T.);
#1984=EDGE_CURVE('',#1575,#1575,#608,.T.);
#1985=EDGE_CURVE('',#1575,#1576,#861,.T.);
#1986=EDGE_CURVE('',#1576,#1576,#609,.T.);
#1987=EDGE_CURVE('',#1577,#1578,#862,.T.);
#1988=EDGE_CURVE('',#1577,#1579,#863,.T.);
#1989=EDGE_CURVE('',#1579,#1580,#864,.T.);
#1990=EDGE_CURVE('',#1578,#1580,#865,.T.);
#1991=EDGE_CURVE('',#1581,#1582,#866,.T.);
#1992=EDGE_CURVE('',#1583,#1581,#867,.T.);
#1993=EDGE_CURVE('',#1583,#1584,#868,.T.);
#1994=EDGE_CURVE('',#1582,#1584,#869,.T.);
#1995=EDGE_CURVE('',#1585,#1586,#870,.T.);
#1996=EDGE_CURVE('',#1586,#1587,#871,.T.);
#1997=EDGE_CURVE('',#1587,#1555,#872,.T.);
#1998=EDGE_CURVE('',#1588,#1554,#873,.T.);
#1999=EDGE_CURVE('',#1588,#1585,#874,.T.);
#2000=EDGE_CURVE('',#1589,#1590,#875,.T.);
#2001=EDGE_CURVE('',#1590,#1591,#876,.T.);
#2002=EDGE_CURVE('',#1549,#1591,#877,.T.);
#2003=EDGE_CURVE('',#1548,#1592,#878,.T.);
#2004=EDGE_CURVE('',#1592,#1589,#879,.T.);
#2005=EDGE_CURVE('',#1593,#1594,#610,.T.);
#2006=EDGE_CURVE('',#1593,#1595,#880,.T.);
#2007=EDGE_CURVE('',#1596,#1595,#611,.T.);
#2008=EDGE_CURVE('',#1597,#1596,#612,.T.);
#2009=EDGE_CURVE('',#1594,#1597,#881,.T.);
#2010=EDGE_CURVE('',#1598,#1599,#613,.T.);
#2011=EDGE_CURVE('',#1599,#1600,#882,.T.);
#2012=EDGE_CURVE('',#1601,#1600,#614,.T.);
#2013=EDGE_CURVE('',#1598,#1601,#883,.T.);
#2014=EDGE_CURVE('',#1599,#1602,#884,.T.);
#2015=EDGE_CURVE('',#1602,#1603,#885,.T.);
#2016=EDGE_CURVE('',#1600,#1603,#886,.T.);
#2017=EDGE_CURVE('',#1604,#1602,#615,.T.);
#2018=EDGE_CURVE('',#1604,#1605,#887,.T.);
#2019=EDGE_CURVE('',#1603,#1605,#616,.T.);
#2020=EDGE_CURVE('',#1606,#1573,#617,.T.);
#2021=EDGE_CURVE('',#1606,#1607,#888,.T.);
#2022=EDGE_CURVE('',#1574,#1607,#618,.T.);
#2023=EDGE_CURVE('',#1608,#1606,#889,.T.);
#2024=EDGE_CURVE('',#1608,#1609,#890,.T.);
#2025=EDGE_CURVE('',#1607,#1609,#891,.T.);
#2026=EDGE_CURVE('',#1610,#1608,#619,.T.);
#2027=EDGE_CURVE('',#1610,#1611,#892,.T.);
#2028=EDGE_CURVE('',#1609,#1611,#620,.T.);
#2029=EDGE_CURVE('',#1591,#1612,#893,.T.);
#2030=EDGE_CURVE('',#1612,#1613,#894,.T.);
#2031=EDGE_CURVE('',#1613,#1614,#895,.T.);
#2032=EDGE_CURVE('',#1615,#1614,#896,.T.);
#2033=EDGE_CURVE('',#1596,#1615,#897,.T.);
#2034=EDGE_CURVE('',#1611,#1596,#898,.T.);
#2035=EDGE_CURVE('',#1570,#1610,#899,.T.);
#2036=EDGE_CURVE('',#1564,#1572,#900,.T.);
#2037=EDGE_CURVE('',#1578,#1568,#901,.T.);
#2038=EDGE_CURVE('',#1580,#1591,#902,.T.);
#2039=EDGE_CURVE('',#1616,#1615,#621,.T.);
#2040=EDGE_CURVE('',#1597,#1616,#903,.T.);
#2041=EDGE_CURVE('',#1582,#1617,#904,.T.);
#2042=EDGE_CURVE('',#1617,#1618,#905,.T.);
#2043=EDGE_CURVE('',#1618,#1616,#906,.T.);
#2044=EDGE_CURVE('',#1614,#1619,#907,.T.);
#2045=EDGE_CURVE('',#1619,#1577,#908,.T.);
#2046=EDGE_CURVE('',#1567,#1581,#909,.T.);
#2047=EDGE_CURVE('',#1613,#1620,#910,.T.);
#2048=EDGE_CURVE('',#1619,#1620,#911,.T.);
#2049=EDGE_CURVE('',#1620,#1579,#912,.T.);
#2050=EDGE_CURVE('',#1617,#1621,#913,.T.);
#2051=EDGE_CURVE('',#1621,#1622,#914,.T.);
#2052=EDGE_CURVE('',#1618,#1622,#915,.T.);
#2053=EDGE_CURVE('',#1623,#1624,#916,.T.);
#2054=EDGE_CURVE('',#1624,#1625,#917,.T.);
#2055=EDGE_CURVE('',#1553,#1625,#918,.T.);
#2056=EDGE_CURVE('',#1552,#1626,#919,.T.);
#2057=EDGE_CURVE('',#1626,#1623,#920,.T.);
#2058=EDGE_CURVE('',#1612,#1550,#921,.T.);
#2059=EDGE_CURVE('',#1627,#1628,#922,.T.);
#2060=EDGE_CURVE('',#1628,#1629,#923,.T.);
#2061=EDGE_CURVE('',#1629,#1551,#924,.T.);
#2062=EDGE_CURVE('',#1612,#1627,#925,.T.);
#2063=EDGE_CURVE('',#1589,#1628,#926,.T.);
#2064=EDGE_CURVE('',#1627,#1590,#927,.T.);
#2065=EDGE_CURVE('',#1592,#1629,#928,.T.);
#2066=EDGE_CURVE('',#1605,#1565,#622,.T.);
#2067=EDGE_CURVE('',#1563,#1604,#623,.T.);
#2068=EDGE_CURVE('',#1566,#1594,#929,.T.);
#2069=EDGE_CURVE('',#1622,#1625,#930,.T.);
#2070=EDGE_CURVE('',#1625,#1588,#931,.T.);
#2071=EDGE_CURVE('',#1588,#1583,#932,.T.);
#2072=EDGE_CURVE('',#1585,#1624,#933,.T.);
#2073=EDGE_CURVE('',#1623,#1586,#934,.T.);
#2074=EDGE_CURVE('',#1587,#1626,#935,.T.);
#2075=EDGE_CURVE('',#1584,#1621,#936,.T.);
#2076=EDGE_CURVE('',#1630,#1631,#937,.T.);
#2077=EDGE_CURVE('',#1632,#1630,#938,.T.);
#2078=EDGE_CURVE('',#1633,#1632,#939,.T.);
#2079=EDGE_CURVE('',#1634,#1633,#940,.T.);
#2080=EDGE_CURVE('',#1635,#1634,#941,.T.);
#2081=EDGE_CURVE('',#1631,#1635,#942,.T.);
#2082=EDGE_CURVE('',#1636,#1637,#943,.T.);
#2083=EDGE_CURVE('',#1638,#1636,#944,.T.);
#2084=EDGE_CURVE('',#1639,#1638,#945,.T.);
#2085=EDGE_CURVE('',#1640,#1639,#946,.T.);
#2086=EDGE_CURVE('',#1641,#1640,#947,.T.);
#2087=EDGE_CURVE('',#1641,#1637,#948,.T.);
#2088=EDGE_CURVE('',#1642,#1636,#949,.T.);
#2089=EDGE_CURVE('',#1643,#1642,#950,.T.);
#2090=EDGE_CURVE('',#1644,#1643,#951,.T.);
#2091=EDGE_CURVE('',#1644,#1638,#952,.T.);
#2092=EDGE_CURVE('',#1645,#1645,#624,.T.);
#2093=EDGE_CURVE('',#1645,#1646,#953,.T.);
#2094=EDGE_CURVE('',#1646,#1646,#625,.T.);
#2095=EDGE_CURVE('',#1647,#1635,#954,.T.);
#2096=EDGE_CURVE('',#1647,#1648,#955,.T.);
#2097=EDGE_CURVE('',#1649,#1648,#956,.T.);
#2098=EDGE_CURVE('',#1649,#1650,#957,.T.);
#2099=EDGE_CURVE('',#1631,#1650,#958,.T.);
#2100=EDGE_CURVE('',#1651,#1652,#959,.T.);
#2101=EDGE_CURVE('',#1651,#1653,#960,.T.);
#2102=EDGE_CURVE('',#1654,#1653,#961,.T.);
#2103=EDGE_CURVE('',#1652,#1654,#962,.T.);
#2104=EDGE_CURVE('',#1652,#1647,#626,.T.);
#2105=EDGE_CURVE('',#1648,#1654,#627,.T.);
#2106=EDGE_CURVE('',#1644,#1655,#628,.T.);
#2107=EDGE_CURVE('',#1650,#1642,#629,.T.);
#2108=EDGE_CURVE('',#1655,#1649,#963,.T.);
#2109=EDGE_CURVE('',#1656,#1655,#964,.T.);
#2110=EDGE_CURVE('',#1657,#1649,#965,.T.);
#2111=EDGE_CURVE('',#1656,#1657,#966,.T.);
#2112=EDGE_CURVE('',#1658,#1639,#967,.T.);
#2113=EDGE_CURVE('',#1658,#1659,#968,.T.);
#2114=EDGE_CURVE('',#1640,#1659,#969,.T.);
#2115=EDGE_CURVE('',#1659,#1660,#970,.T.);
#2116=EDGE_CURVE('',#1641,#1660,#971,.T.);
#2117=EDGE_CURVE('',#1661,#1632,#972,.T.);
#2118=EDGE_CURVE('',#1661,#1662,#973,.T.);
#2119=EDGE_CURVE('',#1662,#1633,#974,.T.);
#2120=EDGE_CURVE('',#1662,#1663,#975,.T.);
#2121=EDGE_CURVE('',#1634,#1663,#976,.T.);
#2122=EDGE_CURVE('',#1598,#1664,#977,.T.);
#2123=EDGE_CURVE('',#1664,#1665,#630,.T.);
#2124=EDGE_CURVE('',#1666,#1665,#978,.T.);
#2125=EDGE_CURVE('',#1666,#1658,#979,.T.);
#2126=EDGE_CURVE('',#1656,#1667,#631,.T.);
#2127=EDGE_CURVE('',#1667,#1668,#980,.T.);
#2128=EDGE_CURVE('',#1668,#1669,#632,.T.);
#2129=EDGE_CURVE('',#1670,#1669,#981,.T.);
#2130=EDGE_CURVE('',#1671,#1670,#633,.T.);
#2131=EDGE_CURVE('',#1593,#1671,#982,.T.);
#2132=EDGE_CURVE('',#1663,#1672,#983,.T.);
#2133=EDGE_CURVE('',#1672,#1673,#984,.T.);
#2134=EDGE_CURVE('',#1673,#1674,#634,.T.);
#2135=EDGE_CURVE('',#1674,#1675,#985,.T.);
#2136=EDGE_CURVE('',#1675,#1651,#635,.T.);
#2137=EDGE_CURVE('',#1676,#1630,#986,.T.);
#2138=EDGE_CURVE('',#1661,#1676,#987,.T.);
#2139=EDGE_CURVE('',#1637,#1677,#988,.T.);
#2140=EDGE_CURVE('',#1677,#1678,#989,.T.);
#2141=EDGE_CURVE('',#1678,#1679,#990,.T.);
#2142=EDGE_CURVE('',#1679,#1680,#636,.T.);
#2143=EDGE_CURVE('',#1680,#1681,#991,.T.);
#2144=EDGE_CURVE('',#1681,#1676,#992,.T.);
#2145=EDGE_CURVE('',#1682,#1601,#993,.T.);
#2146=EDGE_CURVE('',#1664,#1682,#994,.T.);
#2147=EDGE_CURVE('',#1683,#1657,#637,.T.);
#2148=EDGE_CURVE('',#1667,#1683,#995,.T.);
#2149=EDGE_CURVE('',#1595,#1684,#996,.T.);
#2150=EDGE_CURVE('',#1684,#1685,#638,.T.);
#2151=EDGE_CURVE('',#1685,#1686,#997,.T.);
#2152=EDGE_CURVE('',#1686,#1687,#639,.T.);
#2153=EDGE_CURVE('',#1687,#1683,#998,.T.);
#2154=EDGE_CURVE('',#1653,#1688,#640,.T.);
#2155=EDGE_CURVE('',#1688,#1689,#999,.T.);
#2156=EDGE_CURVE('',#1689,#1690,#641,.T.);
#2157=EDGE_CURVE('',#1690,#1691,#1000,.T.);
#2158=EDGE_CURVE('',#1691,#1682,#642,.T.);
#2159=EDGE_CURVE('',#1672,#1681,#1001,.T.);
#2160=EDGE_CURVE('',#1660,#1677,#1002,.T.);
#2161=EDGE_CURVE('',#1678,#1666,#1003,.T.);
#2162=EDGE_CURVE('',#1691,#1680,#1004,.T.);
#2163=EDGE_CURVE('',#1673,#1690,#1005,.T.);
#2164=EDGE_CURVE('',#1674,#1689,#1006,.T.);
#2165=EDGE_CURVE('',#1675,#1688,#1007,.T.);
#2166=EDGE_CURVE('',#1668,#1687,#1008,.T.);
#2167=EDGE_CURVE('',#1669,#1686,#1009,.T.);
#2168=EDGE_CURVE('',#1670,#1685,#1010,.T.);
#2169=EDGE_CURVE('',#1684,#1671,#1011,.T.);
#2170=EDGE_CURVE('',#1665,#1692,#1012,.T.);
#2171=EDGE_CURVE('',#1692,#1679,#1013,.T.);
#2654=ORIENTED_EDGE('',*,*,#1937,.F.);
#2655=ORIENTED_EDGE('',*,*,#1938,.T.);
#2656=ORIENTED_EDGE('',*,*,#1939,.F.);
#2657=ORIENTED_EDGE('',*,*,#1940,.F.);
#2658=ORIENTED_EDGE('',*,*,#1941,.F.);
#2659=ORIENTED_EDGE('',*,*,#1942,.T.);
#2660=ORIENTED_EDGE('',*,*,#1943,.F.);
#2661=ORIENTED_EDGE('',*,*,#1938,.F.);
#2662=ORIENTED_EDGE('',*,*,#1944,.F.);
#2663=ORIENTED_EDGE('',*,*,#1942,.F.);
#2664=ORIENTED_EDGE('',*,*,#1945,.F.);
#2665=ORIENTED_EDGE('',*,*,#1946,.T.);
#2666=ORIENTED_EDGE('',*,*,#1947,.F.);
#2667=ORIENTED_EDGE('',*,*,#1948,.F.);
#2668=ORIENTED_EDGE('',*,*,#1949,.F.);
#2669=ORIENTED_EDGE('',*,*,#1946,.F.);
#2670=ORIENTED_EDGE('',*,*,#1947,.T.);
#2671=ORIENTED_EDGE('',*,*,#1949,.T.);
#2672=ORIENTED_EDGE('',*,*,#1950,.F.);
#2673=ORIENTED_EDGE('',*,*,#1951,.F.);
#2674=ORIENTED_EDGE('',*,*,#1952,.F.);
#2675=ORIENTED_EDGE('',*,*,#1953,.F.);
#2676=ORIENTED_EDGE('',*,*,#1954,.F.);
#2677=ORIENTED_EDGE('',*,*,#1939,.T.);
#2678=ORIENTED_EDGE('',*,*,#1941,.T.);
#2679=ORIENTED_EDGE('',*,*,#1955,.T.);
#2680=ORIENTED_EDGE('',*,*,#1956,.F.);
#2681=ORIENTED_EDGE('',*,*,#1957,.F.);
#2682=ORIENTED_EDGE('',*,*,#1958,.F.);
#2683=ORIENTED_EDGE('',*,*,#1959,.T.);
#2684=ORIENTED_EDGE('',*,*,#1960,.F.);
#2685=ORIENTED_EDGE('',*,*,#1961,.T.);
#2686=ORIENTED_EDGE('',*,*,#1962,.F.);
#2687=ORIENTED_EDGE('',*,*,#1961,.F.);
#2688=ORIENTED_EDGE('',*,*,#1963,.F.);
#2689=ORIENTED_EDGE('',*,*,#1964,.T.);
#2690=ORIENTED_EDGE('',*,*,#1965,.T.);
#2691=ORIENTED_EDGE('',*,*,#1964,.F.);
#2692=ORIENTED_EDGE('',*,*,#1965,.F.);
#2693=ORIENTED_EDGE('',*,*,#1966,.F.);
#2694=ORIENTED_EDGE('',*,*,#1967,.T.);
#2695=ORIENTED_EDGE('',*,*,#1968,.T.);
#2696=ORIENTED_EDGE('',*,*,#1967,.F.);
#2697=ORIENTED_EDGE('',*,*,#1968,.F.);
#2698=ORIENTED_EDGE('',*,*,#1969,.F.);
#2699=ORIENTED_EDGE('',*,*,#1970,.T.);
#2700=ORIENTED_EDGE('',*,*,#1971,.F.);
#2701=ORIENTED_EDGE('',*,*,#1972,.F.);
#2702=ORIENTED_EDGE('',*,*,#1973,.F.);
#2703=ORIENTED_EDGE('',*,*,#1974,.T.);
#2704=ORIENTED_EDGE('',*,*,#1975,.F.);
#2705=ORIENTED_EDGE('',*,*,#1976,.F.);
#2706=ORIENTED_EDGE('',*,*,#1970,.F.);
#2707=ORIENTED_EDGE('',*,*,#1977,.F.);
#2708=ORIENTED_EDGE('',*,*,#1978,.T.);
#2709=ORIENTED_EDGE('',*,*,#1979,.F.);
#2710=ORIENTED_EDGE('',*,*,#1980,.F.);
#2711=ORIENTED_EDGE('',*,*,#1981,.F.);
#2712=ORIENTED_EDGE('',*,*,#1982,.T.);
#2713=ORIENTED_EDGE('',*,*,#1983,.F.);
#2714=ORIENTED_EDGE('',*,*,#1978,.F.);
#2715=ORIENTED_EDGE('',*,*,#1984,.F.);
#2716=ORIENTED_EDGE('',*,*,#1985,.T.);
#2717=ORIENTED_EDGE('',*,*,#1986,.F.);
#2718=ORIENTED_EDGE('',*,*,#1985,.F.);
#2719=ORIENTED_EDGE('',*,*,#1984,.T.);
#2720=ORIENTED_EDGE('',*,*,#1987,.F.);
#2721=ORIENTED_EDGE('',*,*,#1988,.T.);
#2722=ORIENTED_EDGE('',*,*,#1989,.T.);
#2723=ORIENTED_EDGE('',*,*,#1990,.F.);
#2724=ORIENTED_EDGE('',*,*,#1991,.F.);
#2725=ORIENTED_EDGE('',*,*,#1992,.F.);
#2726=ORIENTED_EDGE('',*,*,#1993,.T.);
#2727=ORIENTED_EDGE('',*,*,#1994,.F.);
#2728=ORIENTED_EDGE('',*,*,#1995,.T.);
#2729=ORIENTED_EDGE('',*,*,#1996,.T.);
#2730=ORIENTED_EDGE('',*,*,#1997,.T.);
#2731=ORIENTED_EDGE('',*,*,#1958,.T.);
#2732=ORIENTED_EDGE('',*,*,#1998,.F.);
#2733=ORIENTED_EDGE('',*,*,#1999,.T.);
#2734=ORIENTED_EDGE('',*,*,#2000,.T.);
#2735=ORIENTED_EDGE('',*,*,#2001,.T.);
#2736=ORIENTED_EDGE('',*,*,#2002,.F.);
#2737=ORIENTED_EDGE('',*,*,#1951,.T.);
#2738=ORIENTED_EDGE('',*,*,#2003,.T.);
#2739=ORIENTED_EDGE('',*,*,#2004,.T.);
#2740=ORIENTED_EDGE('',*,*,#2005,.F.);
#2741=ORIENTED_EDGE('',*,*,#2006,.T.);
#2742=ORIENTED_EDGE('',*,*,#2007,.F.);
#2743=ORIENTED_EDGE('',*,*,#2008,.F.);
#2744=ORIENTED_EDGE('',*,*,#2009,.F.);
#2745=ORIENTED_EDGE('',*,*,#2010,.T.);
#2746=ORIENTED_EDGE('',*,*,#2011,.T.);
#2747=ORIENTED_EDGE('',*,*,#2012,.F.);
#2748=ORIENTED_EDGE('',*,*,#2013,.F.);
#2749=ORIENTED_EDGE('',*,*,#2014,.T.);
#2750=ORIENTED_EDGE('',*,*,#2015,.T.);
#2751=ORIENTED_EDGE('',*,*,#2016,.F.);
#2752=ORIENTED_EDGE('',*,*,#2011,.F.);
#2753=ORIENTED_EDGE('',*,*,#2017,.F.);
#2754=ORIENTED_EDGE('',*,*,#2018,.T.);
#2755=ORIENTED_EDGE('',*,*,#2019,.F.);
#2756=ORIENTED_EDGE('',*,*,#2015,.F.);
#2757=ORIENTED_EDGE('',*,*,#2020,.F.);
#2758=ORIENTED_EDGE('',*,*,#2021,.T.);
#2759=ORIENTED_EDGE('',*,*,#2022,.F.);
#2760=ORIENTED_EDGE('',*,*,#1982,.F.);
#2761=ORIENTED_EDGE('',*,*,#2023,.F.);
#2762=ORIENTED_EDGE('',*,*,#2024,.T.);
#2763=ORIENTED_EDGE('',*,*,#2025,.F.);
#2764=ORIENTED_EDGE('',*,*,#2021,.F.);
#2765=ORIENTED_EDGE('',*,*,#2026,.F.);
#2766=ORIENTED_EDGE('',*,*,#2027,.T.);
#2767=ORIENTED_EDGE('',*,*,#2028,.F.);
#2768=ORIENTED_EDGE('',*,*,#2024,.F.);
#2769=ORIENTED_EDGE('',*,*,#2029,.T.);
#2770=ORIENTED_EDGE('',*,*,#2030,.T.);
#2771=ORIENTED_EDGE('',*,*,#2031,.T.);
#2772=ORIENTED_EDGE('',*,*,#2032,.F.);
#2773=ORIENTED_EDGE('',*,*,#2033,.F.);
#2774=ORIENTED_EDGE('',*,*,#2034,.F.);
#2775=ORIENTED_EDGE('',*,*,#2027,.F.);
#2776=ORIENTED_EDGE('',*,*,#2035,.F.);
#2777=ORIENTED_EDGE('',*,*,#1980,.T.);
#2778=ORIENTED_EDGE('',*,*,#2036,.F.);
#2779=ORIENTED_EDGE('',*,*,#1976,.T.);
#2780=ORIENTED_EDGE('',*,*,#2037,.F.);
#2781=ORIENTED_EDGE('',*,*,#1990,.T.);
#2782=ORIENTED_EDGE('',*,*,#2038,.T.);
#2783=ORIENTED_EDGE('',*,*,#2008,.T.);
#2784=ORIENTED_EDGE('',*,*,#2033,.T.);
#2785=ORIENTED_EDGE('',*,*,#2039,.F.);
#2786=ORIENTED_EDGE('',*,*,#2040,.F.);
#2787=ORIENTED_EDGE('',*,*,#2041,.T.);
#2788=ORIENTED_EDGE('',*,*,#2042,.T.);
#2789=ORIENTED_EDGE('',*,*,#2043,.T.);
#2790=ORIENTED_EDGE('',*,*,#2039,.T.);
#2791=ORIENTED_EDGE('',*,*,#2032,.T.);
#2792=ORIENTED_EDGE('',*,*,#2044,.T.);
#2793=ORIENTED_EDGE('',*,*,#2045,.T.);
#2794=ORIENTED_EDGE('',*,*,#1987,.T.);
#2795=ORIENTED_EDGE('',*,*,#2037,.T.);
#2796=ORIENTED_EDGE('',*,*,#1975,.T.);
#2797=ORIENTED_EDGE('',*,*,#2046,.T.);
#2798=ORIENTED_EDGE('',*,*,#1991,.T.);
#2799=ORIENTED_EDGE('',*,*,#1986,.T.);
#2800=ORIENTED_EDGE('',*,*,#1963,.T.);
#2801=ORIENTED_EDGE('',*,*,#2044,.F.);
#2802=ORIENTED_EDGE('',*,*,#2031,.F.);
#2803=ORIENTED_EDGE('',*,*,#2047,.T.);
#2804=ORIENTED_EDGE('',*,*,#2048,.F.);
#2805=ORIENTED_EDGE('',*,*,#2045,.F.);
#2806=ORIENTED_EDGE('',*,*,#2048,.T.);
#2807=ORIENTED_EDGE('',*,*,#2049,.T.);
#2808=ORIENTED_EDGE('',*,*,#1988,.F.);
#2809=ORIENTED_EDGE('',*,*,#2042,.F.);
#2810=ORIENTED_EDGE('',*,*,#2050,.T.);
#2811=ORIENTED_EDGE('',*,*,#2051,.T.);
#2812=ORIENTED_EDGE('',*,*,#2052,.F.);
#2813=ORIENTED_EDGE('',*,*,#2053,.T.);
#2814=ORIENTED_EDGE('',*,*,#2054,.T.);
#2815=ORIENTED_EDGE('',*,*,#2055,.F.);
#2816=ORIENTED_EDGE('',*,*,#1956,.T.);
#2817=ORIENTED_EDGE('',*,*,#2056,.T.);
#2818=ORIENTED_EDGE('',*,*,#2057,.T.);
#2819=ORIENTED_EDGE('',*,*,#2049,.F.);
#2820=ORIENTED_EDGE('',*,*,#2047,.F.);
#2821=ORIENTED_EDGE('',*,*,#2030,.F.);
#2822=ORIENTED_EDGE('',*,*,#2058,.T.);
#2823=ORIENTED_EDGE('',*,*,#1952,.T.);
#2824=ORIENTED_EDGE('',*,*,#2002,.T.);
#2825=ORIENTED_EDGE('',*,*,#2038,.F.);
#2826=ORIENTED_EDGE('',*,*,#1989,.F.);
#2827=ORIENTED_EDGE('',*,*,#2059,.T.);
#2828=ORIENTED_EDGE('',*,*,#2060,.T.);
#2829=ORIENTED_EDGE('',*,*,#2061,.T.);
#2830=ORIENTED_EDGE('',*,*,#1953,.T.);
#2831=ORIENTED_EDGE('',*,*,#2058,.F.);
#2832=ORIENTED_EDGE('',*,*,#2062,.T.);
#2833=ORIENTED_EDGE('',*,*,#2063,.T.);
#2834=ORIENTED_EDGE('',*,*,#2059,.F.);
#2835=ORIENTED_EDGE('',*,*,#2064,.T.);
#2836=ORIENTED_EDGE('',*,*,#2000,.F.);
#2837=ORIENTED_EDGE('',*,*,#2065,.T.);
#2838=ORIENTED_EDGE('',*,*,#2060,.F.);
#2839=ORIENTED_EDGE('',*,*,#2063,.F.);
#2840=ORIENTED_EDGE('',*,*,#2004,.F.);
#2841=ORIENTED_EDGE('',*,*,#1948,.T.);
#2842=ORIENTED_EDGE('',*,*,#1954,.T.);
#2843=ORIENTED_EDGE('',*,*,#2061,.F.);
#2844=ORIENTED_EDGE('',*,*,#2065,.F.);
#2845=ORIENTED_EDGE('',*,*,#2003,.F.);
#2846=ORIENTED_EDGE('',*,*,#1950,.T.);
#2847=ORIENTED_EDGE('',*,*,#2064,.F.);
#2848=ORIENTED_EDGE('',*,*,#2062,.F.);
#2849=ORIENTED_EDGE('',*,*,#2029,.F.);
#2850=ORIENTED_EDGE('',*,*,#2001,.F.);
#2851=ORIENTED_EDGE('',*,*,#1945,.T.);
#2852=ORIENTED_EDGE('',*,*,#2066,.F.);
#2853=ORIENTED_EDGE('',*,*,#2018,.F.);
#2854=ORIENTED_EDGE('',*,*,#2067,.F.);
#2855=ORIENTED_EDGE('',*,*,#1972,.T.);
#2856=ORIENTED_EDGE('',*,*,#2068,.T.);
#2857=ORIENTED_EDGE('',*,*,#2009,.T.);
#2858=ORIENTED_EDGE('',*,*,#2040,.T.);
#2859=ORIENTED_EDGE('',*,*,#2043,.F.);
#2860=ORIENTED_EDGE('',*,*,#2052,.T.);
#2861=ORIENTED_EDGE('',*,*,#2069,.T.);
#2862=ORIENTED_EDGE('',*,*,#2070,.T.);
#2863=ORIENTED_EDGE('',*,*,#2071,.T.);
#2864=ORIENTED_EDGE('',*,*,#1992,.T.);
#2865=ORIENTED_EDGE('',*,*,#2046,.F.);
#2866=ORIENTED_EDGE('',*,*,#1974,.F.);
#2867=ORIENTED_EDGE('',*,*,#2070,.F.);
#2868=ORIENTED_EDGE('',*,*,#2054,.F.);
#2869=ORIENTED_EDGE('',*,*,#2072,.F.);
#2870=ORIENTED_EDGE('',*,*,#1999,.F.);
#2871=ORIENTED_EDGE('',*,*,#1943,.T.);
#2872=ORIENTED_EDGE('',*,*,#1944,.T.);
#2873=ORIENTED_EDGE('',*,*,#1937,.T.);
#2874=ORIENTED_EDGE('',*,*,#2072,.T.);
#2875=ORIENTED_EDGE('',*,*,#2053,.F.);
#2876=ORIENTED_EDGE('',*,*,#2073,.T.);
#2877=ORIENTED_EDGE('',*,*,#1995,.F.);
#2878=ORIENTED_EDGE('',*,*,#2073,.F.);
#2879=ORIENTED_EDGE('',*,*,#2057,.F.);
#2880=ORIENTED_EDGE('',*,*,#2074,.F.);
#2881=ORIENTED_EDGE('',*,*,#1996,.F.);
#2882=ORIENTED_EDGE('',*,*,#1940,.T.);
#2883=ORIENTED_EDGE('',*,*,#1959,.F.);
#2884=ORIENTED_EDGE('',*,*,#1997,.F.);
#2885=ORIENTED_EDGE('',*,*,#2074,.T.);
#2886=ORIENTED_EDGE('',*,*,#2056,.F.);
#2887=ORIENTED_EDGE('',*,*,#1955,.F.);
#2888=ORIENTED_EDGE('',*,*,#1957,.T.);
#2889=ORIENTED_EDGE('',*,*,#2055,.T.);
#2890=ORIENTED_EDGE('',*,*,#2069,.F.);
#2891=ORIENTED_EDGE('',*,*,#2051,.F.);
#2892=ORIENTED_EDGE('',*,*,#2075,.F.);
#2893=ORIENTED_EDGE('',*,*,#1993,.F.);
#2894=ORIENTED_EDGE('',*,*,#2071,.F.);
#2895=ORIENTED_EDGE('',*,*,#1998,.T.);
#2896=ORIENTED_EDGE('',*,*,#2075,.T.);
#2897=ORIENTED_EDGE('',*,*,#2050,.F.);
#2898=ORIENTED_EDGE('',*,*,#2041,.F.);
#2899=ORIENTED_EDGE('',*,*,#1994,.T.);
#2900=ORIENTED_EDGE('',*,*,#2076,.F.);
#2901=ORIENTED_EDGE('',*,*,#2077,.F.);
#2902=ORIENTED_EDGE('',*,*,#2078,.F.);
#2903=ORIENTED_EDGE('',*,*,#2079,.F.);
#2904=ORIENTED_EDGE('',*,*,#2080,.F.);
#2905=ORIENTED_EDGE('',*,*,#2081,.F.);
#2906=ORIENTED_EDGE('',*,*,#2082,.F.);
#2907=ORIENTED_EDGE('',*,*,#2083,.F.);
#2908=ORIENTED_EDGE('',*,*,#2084,.F.);
#2909=ORIENTED_EDGE('',*,*,#2085,.F.);
#2910=ORIENTED_EDGE('',*,*,#2086,.F.);
#2911=ORIENTED_EDGE('',*,*,#2087,.T.);
#2912=ORIENTED_EDGE('',*,*,#2083,.T.);
#2913=ORIENTED_EDGE('',*,*,#2088,.F.);
#2914=ORIENTED_EDGE('',*,*,#2089,.F.);
#2915=ORIENTED_EDGE('',*,*,#2090,.F.);
#2916=ORIENTED_EDGE('',*,*,#2091,.T.);
#2917=ORIENTED_EDGE('',*,*,#2092,.T.);
#2918=ORIENTED_EDGE('',*,*,#2092,.F.);
#2919=ORIENTED_EDGE('',*,*,#2093,.T.);
#2920=ORIENTED_EDGE('',*,*,#2094,.F.);
#2921=ORIENTED_EDGE('',*,*,#2093,.F.);
#2922=ORIENTED_EDGE('',*,*,#2081,.T.);
#2923=ORIENTED_EDGE('',*,*,#2095,.F.);
#2924=ORIENTED_EDGE('',*,*,#2096,.T.);
#2925=ORIENTED_EDGE('',*,*,#2097,.F.);
#2926=ORIENTED_EDGE('',*,*,#2098,.T.);
#2927=ORIENTED_EDGE('',*,*,#2099,.F.);
#2928=ORIENTED_EDGE('',*,*,#2100,.F.);
#2929=ORIENTED_EDGE('',*,*,#2101,.T.);
#2930=ORIENTED_EDGE('',*,*,#2102,.F.);
#2931=ORIENTED_EDGE('',*,*,#2103,.F.);
#2932=ORIENTED_EDGE('',*,*,#2104,.F.);
#2933=ORIENTED_EDGE('',*,*,#2103,.T.);
#2934=ORIENTED_EDGE('',*,*,#2105,.F.);
#2935=ORIENTED_EDGE('',*,*,#2096,.F.);
#2936=ORIENTED_EDGE('',*,*,#2106,.F.);
#2937=ORIENTED_EDGE('',*,*,#2090,.T.);
#2938=ORIENTED_EDGE('',*,*,#2089,.T.);
#2939=ORIENTED_EDGE('',*,*,#2107,.F.);
#2940=ORIENTED_EDGE('',*,*,#2098,.F.);
#2941=ORIENTED_EDGE('',*,*,#2108,.F.);
#2942=ORIENTED_EDGE('',*,*,#2109,.T.);
#2943=ORIENTED_EDGE('',*,*,#2108,.T.);
#2944=ORIENTED_EDGE('',*,*,#2110,.F.);
#2945=ORIENTED_EDGE('',*,*,#2111,.F.);
#2946=ORIENTED_EDGE('',*,*,#2112,.F.);
#2947=ORIENTED_EDGE('',*,*,#2113,.T.);
#2948=ORIENTED_EDGE('',*,*,#2114,.F.);
#2949=ORIENTED_EDGE('',*,*,#2085,.T.);
#2950=ORIENTED_EDGE('',*,*,#2114,.T.);
#2951=ORIENTED_EDGE('',*,*,#2115,.T.);
#2952=ORIENTED_EDGE('',*,*,#2116,.F.);
#2953=ORIENTED_EDGE('',*,*,#2086,.T.);
#2954=ORIENTED_EDGE('',*,*,#2117,.F.);
#2955=ORIENTED_EDGE('',*,*,#2118,.T.);
#2956=ORIENTED_EDGE('',*,*,#2119,.T.);
#2957=ORIENTED_EDGE('',*,*,#2078,.T.);
#2958=ORIENTED_EDGE('',*,*,#2119,.F.);
#2959=ORIENTED_EDGE('',*,*,#2120,.T.);
#2960=ORIENTED_EDGE('',*,*,#2121,.F.);
#2961=ORIENTED_EDGE('',*,*,#2079,.T.);
#2962=ORIENTED_EDGE('',*,*,#2067,.T.);
#2963=ORIENTED_EDGE('',*,*,#2017,.T.);
#2964=ORIENTED_EDGE('',*,*,#2014,.F.);
#2965=ORIENTED_EDGE('',*,*,#2010,.F.);
#2966=ORIENTED_EDGE('',*,*,#2122,.T.);
#2967=ORIENTED_EDGE('',*,*,#2123,.T.);
#2968=ORIENTED_EDGE('',*,*,#2124,.F.);
#2969=ORIENTED_EDGE('',*,*,#2125,.T.);
#2970=ORIENTED_EDGE('',*,*,#2112,.T.);
#2971=ORIENTED_EDGE('',*,*,#2084,.T.);
#2972=ORIENTED_EDGE('',*,*,#2091,.F.);
#2973=ORIENTED_EDGE('',*,*,#2106,.T.);
#2974=ORIENTED_EDGE('',*,*,#2109,.F.);
#2975=ORIENTED_EDGE('',*,*,#2126,.T.);
#2976=ORIENTED_EDGE('',*,*,#2127,.T.);
#2977=ORIENTED_EDGE('',*,*,#2128,.T.);
#2978=ORIENTED_EDGE('',*,*,#2129,.F.);
#2979=ORIENTED_EDGE('',*,*,#2130,.F.);
#2980=ORIENTED_EDGE('',*,*,#2131,.F.);
#2981=ORIENTED_EDGE('',*,*,#2005,.T.);
#2982=ORIENTED_EDGE('',*,*,#2068,.F.);
#2983=ORIENTED_EDGE('',*,*,#1973,.T.);
#2984=ORIENTED_EDGE('',*,*,#1969,.T.);
#2985=ORIENTED_EDGE('',*,*,#2121,.T.);
#2986=ORIENTED_EDGE('',*,*,#2132,.T.);
#2987=ORIENTED_EDGE('',*,*,#2133,.T.);
#2988=ORIENTED_EDGE('',*,*,#2134,.T.);
#2989=ORIENTED_EDGE('',*,*,#2135,.T.);
#2990=ORIENTED_EDGE('',*,*,#2136,.T.);
#2991=ORIENTED_EDGE('',*,*,#2100,.T.);
#2992=ORIENTED_EDGE('',*,*,#2104,.T.);
#2993=ORIENTED_EDGE('',*,*,#2095,.T.);
#2994=ORIENTED_EDGE('',*,*,#2080,.T.);
#2995=ORIENTED_EDGE('',*,*,#2020,.T.);
#2996=ORIENTED_EDGE('',*,*,#1981,.T.);
#2997=ORIENTED_EDGE('',*,*,#1977,.T.);
#2998=ORIENTED_EDGE('',*,*,#2035,.T.);
#2999=ORIENTED_EDGE('',*,*,#2026,.T.);
#3000=ORIENTED_EDGE('',*,*,#2023,.T.);
#3001=ORIENTED_EDGE('',*,*,#2117,.T.);
#3002=ORIENTED_EDGE('',*,*,#2077,.T.);
#3003=ORIENTED_EDGE('',*,*,#2137,.F.);
#3004=ORIENTED_EDGE('',*,*,#2138,.F.);
#3005=ORIENTED_EDGE('',*,*,#1962,.T.);
#3006=ORIENTED_EDGE('',*,*,#2139,.T.);
#3007=ORIENTED_EDGE('',*,*,#2140,.T.);
#3008=ORIENTED_EDGE('',*,*,#2141,.T.);
#3009=ORIENTED_EDGE('',*,*,#2142,.T.);
#3010=ORIENTED_EDGE('',*,*,#2143,.T.);
#3011=ORIENTED_EDGE('',*,*,#2144,.T.);
#3012=ORIENTED_EDGE('',*,*,#2137,.T.);
#3013=ORIENTED_EDGE('',*,*,#2076,.T.);
#3014=ORIENTED_EDGE('',*,*,#2099,.T.);
#3015=ORIENTED_EDGE('',*,*,#2107,.T.);
#3016=ORIENTED_EDGE('',*,*,#2088,.T.);
#3017=ORIENTED_EDGE('',*,*,#2082,.T.);
#3018=ORIENTED_EDGE('',*,*,#2094,.T.);
#3019=ORIENTED_EDGE('',*,*,#1966,.T.);
#3020=ORIENTED_EDGE('',*,*,#2145,.F.);
#3021=ORIENTED_EDGE('',*,*,#2146,.F.);
#3022=ORIENTED_EDGE('',*,*,#2122,.F.);
#3023=ORIENTED_EDGE('',*,*,#2013,.T.);
#3024=ORIENTED_EDGE('',*,*,#2147,.F.);
#3025=ORIENTED_EDGE('',*,*,#2148,.F.);
#3026=ORIENTED_EDGE('',*,*,#2126,.F.);
#3027=ORIENTED_EDGE('',*,*,#2111,.T.);
#3028=ORIENTED_EDGE('',*,*,#2149,.T.);
#3029=ORIENTED_EDGE('',*,*,#2150,.T.);
#3030=ORIENTED_EDGE('',*,*,#2151,.T.);
#3031=ORIENTED_EDGE('',*,*,#2152,.T.);
#3032=ORIENTED_EDGE('',*,*,#2153,.T.);
#3033=ORIENTED_EDGE('',*,*,#2147,.T.);
#3034=ORIENTED_EDGE('',*,*,#2110,.T.);
#3035=ORIENTED_EDGE('',*,*,#2097,.T.);
#3036=ORIENTED_EDGE('',*,*,#2105,.T.);
#3037=ORIENTED_EDGE('',*,*,#2102,.T.);
#3038=ORIENTED_EDGE('',*,*,#2154,.T.);
#3039=ORIENTED_EDGE('',*,*,#2155,.T.);
#3040=ORIENTED_EDGE('',*,*,#2156,.T.);
#3041=ORIENTED_EDGE('',*,*,#2157,.T.);
#3042=ORIENTED_EDGE('',*,*,#2158,.T.);
#3043=ORIENTED_EDGE('',*,*,#2145,.T.);
#3044=ORIENTED_EDGE('',*,*,#2012,.T.);
#3045=ORIENTED_EDGE('',*,*,#2016,.T.);
#3046=ORIENTED_EDGE('',*,*,#2019,.T.);
#3047=ORIENTED_EDGE('',*,*,#2066,.T.);
#3048=ORIENTED_EDGE('',*,*,#1971,.T.);
#3049=ORIENTED_EDGE('',*,*,#2036,.T.);
#3050=ORIENTED_EDGE('',*,*,#1979,.T.);
#3051=ORIENTED_EDGE('',*,*,#1983,.T.);
#3052=ORIENTED_EDGE('',*,*,#2022,.T.);
#3053=ORIENTED_EDGE('',*,*,#2025,.T.);
#3054=ORIENTED_EDGE('',*,*,#2028,.T.);
#3055=ORIENTED_EDGE('',*,*,#2034,.T.);
#3056=ORIENTED_EDGE('',*,*,#2007,.T.);
#3057=ORIENTED_EDGE('',*,*,#2144,.F.);
#3058=ORIENTED_EDGE('',*,*,#2159,.F.);
#3059=ORIENTED_EDGE('',*,*,#2132,.F.);
#3060=ORIENTED_EDGE('',*,*,#2120,.F.);
#3061=ORIENTED_EDGE('',*,*,#2118,.F.);
#3062=ORIENTED_EDGE('',*,*,#2138,.T.);
#3063=ORIENTED_EDGE('',*,*,#2116,.T.);
#3064=ORIENTED_EDGE('',*,*,#2160,.T.);
#3065=ORIENTED_EDGE('',*,*,#2139,.F.);
#3066=ORIENTED_EDGE('',*,*,#2087,.F.);
#3067=ORIENTED_EDGE('',*,*,#1960,.T.);
#3068=ORIENTED_EDGE('',*,*,#2140,.F.);
#3069=ORIENTED_EDGE('',*,*,#2160,.F.);
#3070=ORIENTED_EDGE('',*,*,#2115,.F.);
#3071=ORIENTED_EDGE('',*,*,#2113,.F.);
#3072=ORIENTED_EDGE('',*,*,#2125,.F.);
#3073=ORIENTED_EDGE('',*,*,#2161,.F.);
#3074=ORIENTED_EDGE('',*,*,#2159,.T.);
#3075=ORIENTED_EDGE('',*,*,#2143,.F.);
#3076=ORIENTED_EDGE('',*,*,#2162,.F.);
#3077=ORIENTED_EDGE('',*,*,#2157,.F.);
#3078=ORIENTED_EDGE('',*,*,#2163,.F.);
#3079=ORIENTED_EDGE('',*,*,#2133,.F.);
#3080=ORIENTED_EDGE('',*,*,#2134,.F.);
#3081=ORIENTED_EDGE('',*,*,#2163,.T.);
#3082=ORIENTED_EDGE('',*,*,#2156,.F.);
#3083=ORIENTED_EDGE('',*,*,#2164,.F.);
#3084=ORIENTED_EDGE('',*,*,#2135,.F.);
#3085=ORIENTED_EDGE('',*,*,#2164,.T.);
#3086=ORIENTED_EDGE('',*,*,#2155,.F.);
#3087=ORIENTED_EDGE('',*,*,#2165,.F.);
#3088=ORIENTED_EDGE('',*,*,#2136,.F.);
#3089=ORIENTED_EDGE('',*,*,#2165,.T.);
#3090=ORIENTED_EDGE('',*,*,#2154,.F.);
#3091=ORIENTED_EDGE('',*,*,#2101,.F.);
#3092=ORIENTED_EDGE('',*,*,#2127,.F.);
#3093=ORIENTED_EDGE('',*,*,#2148,.T.);
#3094=ORIENTED_EDGE('',*,*,#2153,.F.);
#3095=ORIENTED_EDGE('',*,*,#2166,.F.);
#3096=ORIENTED_EDGE('',*,*,#2128,.F.);
#3097=ORIENTED_EDGE('',*,*,#2166,.T.);
#3098=ORIENTED_EDGE('',*,*,#2152,.F.);
#3099=ORIENTED_EDGE('',*,*,#2167,.F.);
#3100=ORIENTED_EDGE('',*,*,#2129,.T.);
#3101=ORIENTED_EDGE('',*,*,#2167,.T.);
#3102=ORIENTED_EDGE('',*,*,#2151,.F.);
#3103=ORIENTED_EDGE('',*,*,#2168,.F.);
#3104=ORIENTED_EDGE('',*,*,#2130,.T.);
#3105=ORIENTED_EDGE('',*,*,#2168,.T.);
#3106=ORIENTED_EDGE('',*,*,#2150,.F.);
#3107=ORIENTED_EDGE('',*,*,#2169,.T.);
#3108=ORIENTED_EDGE('',*,*,#2161,.T.);
#3109=ORIENTED_EDGE('',*,*,#2124,.T.);
#3110=ORIENTED_EDGE('',*,*,#2170,.T.);
#3111=ORIENTED_EDGE('',*,*,#2171,.T.);
#3112=ORIENTED_EDGE('',*,*,#2141,.F.);
#3113=ORIENTED_EDGE('',*,*,#2123,.F.);
#3114=ORIENTED_EDGE('',*,*,#2146,.T.);
#3115=ORIENTED_EDGE('',*,*,#2158,.F.);
#3116=ORIENTED_EDGE('',*,*,#2162,.T.);
#3117=ORIENTED_EDGE('',*,*,#2142,.F.);
#3118=ORIENTED_EDGE('',*,*,#2171,.F.);
#3119=ORIENTED_EDGE('',*,*,#2170,.F.);
#3120=ORIENTED_EDGE('',*,*,#2131,.T.);
#3121=ORIENTED_EDGE('',*,*,#2169,.F.);
#3122=ORIENTED_EDGE('',*,*,#2149,.F.);
#3123=ORIENTED_EDGE('',*,*,#2006,.F.);
#3218=PLANE('',#3705);
#3219=PLANE('',#3718);
#3220=PLANE('',#3719);
#3221=PLANE('',#3726);
#3222=PLANE('',#3730);
#3223=PLANE('',#3731);
#3224=PLANE('',#3738);
#3225=PLANE('',#3742);
#3226=PLANE('',#3743);
#3227=PLANE('',#3744);
#3228=PLANE('',#3745);
#3229=PLANE('',#3746);
#3230=PLANE('',#3754);
#3231=PLANE('',#3761);
#3232=PLANE('',#3765);
#3233=PLANE('',#3768);
#3234=PLANE('',#3769);
#3235=PLANE('',#3770);
#3236=PLANE('',#3771);
#3237=PLANE('',#3772);
#3238=PLANE('',#3773);
#3239=PLANE('',#3774);
#3240=PLANE('',#3775);
#3241=PLANE('',#3776);
#3242=PLANE('',#3777);
#3243=PLANE('',#3778);
#3244=PLANE('',#3782);
#3245=PLANE('',#3783);
#3246=PLANE('',#3784);
#3247=PLANE('',#3785);
#3248=PLANE('',#3786);
#3249=PLANE('',#3787);
#3250=PLANE('',#3788);
#3251=PLANE('',#3789);
#3252=PLANE('',#3790);
#3253=PLANE('',#3791);
#3254=PLANE('',#3792);
#3255=PLANE('',#3796);
#3256=PLANE('',#3797);
#3257=PLANE('',#3804);
#3258=PLANE('',#3805);
#3259=PLANE('',#3806);
#3260=PLANE('',#3807);
#3261=PLANE('',#3808);
#3262=PLANE('',#3809);
#3263=PLANE('',#3816);
#3264=PLANE('',#3817);
#3265=PLANE('',#3819);
#3266=PLANE('',#3822);
#3267=PLANE('',#3828);
#3268=PLANE('',#3829);
#3269=PLANE('',#3830);
#3270=PLANE('',#3831);
#3271=PLANE('',#3833);
#3272=PLANE('',#3835);
#3273=PLANE('',#3837);
#3274=PLANE('',#3839);
#3275=PLANE('',#3841);
#3370=ADVANCED_FACE('',(#250),#3218,.T.);
#3371=ADVANCED_FACE('',(#251),#138,.F.);
#3372=ADVANCED_FACE('',(#252),#139,.F.);
#3373=ADVANCED_FACE('',(#253),#3219,.T.);
#3374=ADVANCED_FACE('',(#254),#3220,.T.);
#3375=ADVANCED_FACE('',(#255),#140,.F.);
#3376=ADVANCED_FACE('',(#256),#141,.F.);
#3377=ADVANCED_FACE('',(#257),#3221,.T.);
#3378=ADVANCED_FACE('',(#258),#142,.F.);
#3379=ADVANCED_FACE('',(#259),#3222,.T.);
#3380=ADVANCED_FACE('',(#260),#3223,.T.);
#3381=ADVANCED_FACE('',(#261),#143,.T.);
#3382=ADVANCED_FACE('',(#262),#144,.F.);
#3383=ADVANCED_FACE('',(#263),#3224,.T.);
#3384=ADVANCED_FACE('',(#264),#145,.F.);
#3385=ADVANCED_FACE('',(#265),#3225,.F.);
#3386=ADVANCED_FACE('',(#266),#3226,.F.);
#3387=ADVANCED_FACE('',(#267),#3227,.F.);
#3388=ADVANCED_FACE('',(#268),#3228,.T.);
#3389=ADVANCED_FACE('',(#269),#3229,.T.);
#3390=ADVANCED_FACE('',(#270),#146,.T.);
#3391=ADVANCED_FACE('',(#271),#147,.F.);
#3392=ADVANCED_FACE('',(#272),#3230,.T.);
#3393=ADVANCED_FACE('',(#273),#148,.T.);
#3394=ADVANCED_FACE('',(#274),#149,.F.);
#3395=ADVANCED_FACE('',(#275),#3231,.T.);
#3396=ADVANCED_FACE('',(#276),#150,.F.);
#3397=ADVANCED_FACE('',(#277),#3232,.T.);
#3398=ADVANCED_FACE('',(#278),#151,.T.);
#3399=ADVANCED_FACE('',(#279,#86,#87),#3233,.F.);
#3400=ADVANCED_FACE('',(#280),#3234,.F.);
#3401=ADVANCED_FACE('',(#281),#3235,.F.);
#3402=ADVANCED_FACE('',(#282),#3236,.F.);
#3403=ADVANCED_FACE('',(#283),#3237,.T.);
#3404=ADVANCED_FACE('',(#284),#3238,.F.);
#3405=ADVANCED_FACE('',(#285),#3239,.T.);
#3406=ADVANCED_FACE('',(#286),#3240,.T.);
#3407=ADVANCED_FACE('',(#287),#3241,.T.);
#3408=ADVANCED_FACE('',(#288),#3242,.T.);
#3409=ADVANCED_FACE('',(#289,#88),#3243,.T.);
#3410=ADVANCED_FACE('',(#290),#152,.T.);
#3411=ADVANCED_FACE('',(#291),#3244,.T.);
#3412=ADVANCED_FACE('',(#292,#89),#3245,.T.);
#3413=ADVANCED_FACE('',(#293),#3246,.T.);
#3414=ADVANCED_FACE('',(#294),#3247,.T.);
#3415=ADVANCED_FACE('',(#295),#3248,.T.);
#3416=ADVANCED_FACE('',(#296),#3249,.F.);
#3417=ADVANCED_FACE('',(#297),#3250,.F.);
#3418=ADVANCED_FACE('',(#298),#3251,.F.);
#3419=ADVANCED_FACE('',(#299),#3252,.F.);
#3420=ADVANCED_FACE('',(#300),#3253,.T.);
#3421=ADVANCED_FACE('',(#301),#3254,.F.);
#3422=ADVANCED_FACE('',(#302),#153,.F.);
#3423=ADVANCED_FACE('',(#303),#3255,.T.);
#3424=ADVANCED_FACE('',(#304),#3256,.T.);
#3425=ADVANCED_FACE('',(#305),#154,.F.);
#3426=ADVANCED_FACE('',(#306),#155,.T.);
#3427=ADVANCED_FACE('',(#307),#3257,.T.);
#3428=ADVANCED_FACE('',(#308),#3258,.F.);
#3429=ADVANCED_FACE('',(#309),#3259,.F.);
#3430=ADVANCED_FACE('',(#310),#3260,.F.);
#3431=ADVANCED_FACE('',(#311),#3261,.F.);
#3432=ADVANCED_FACE('',(#312,#90,#91),#3262,.T.);
#3433=ADVANCED_FACE('',(#313,#92),#3263,.F.);
#3434=ADVANCED_FACE('',(#314,#93,#94),#3264,.F.);
#3435=ADVANCED_FACE('',(#315),#3265,.T.);
#3436=ADVANCED_FACE('',(#316),#156,.T.);
#3437=ADVANCED_FACE('',(#317),#3266,.F.);
#3438=ADVANCED_FACE('',(#318),#3267,.F.);
#3439=ADVANCED_FACE('',(#319,#95),#3268,.F.);
#3440=ADVANCED_FACE('',(#320),#3269,.F.);
#3441=ADVANCED_FACE('',(#321),#3270,.T.);
#3442=ADVANCED_FACE('',(#322),#157,.F.);
#3443=ADVANCED_FACE('',(#323),#3271,.T.);
#3444=ADVANCED_FACE('',(#324),#158,.F.);
#3445=ADVANCED_FACE('',(#325),#3272,.T.);
#3446=ADVANCED_FACE('',(#326),#159,.T.);
#3447=ADVANCED_FACE('',(#327),#3273,.T.);
#3448=ADVANCED_FACE('',(#328),#160,.F.);
#3449=ADVANCED_FACE('',(#329),#3274,.T.);
#3450=ADVANCED_FACE('',(#330),#161,.T.);
#3451=ADVANCED_FACE('',(#331),#3275,.T.);
#3471=CLOSED_SHELL('',(#3370,#3371,#3372,#3373,#3374,#3375,#3376,#3377,
#3378,#3379,#3380,#3381,#3382,#3383,#3384,#3385,#3386,#3387,#3388,#3389,
#3390,#3391,#3392,#3393,#3394,#3395,#3396,#3397,#3398,#3399,#3400,#3401,
#3402,#3403,#3404,#3405,#3406,#3407,#3408,#3409,#3410,#3411,#3412,#3413,
#3414,#3415,#3416,#3417,#3418,#3419,#3420,#3421,#3422,#3423,#3424,#3425,
#3426,#3427,#3428,#3429,#3430,#3431,#3432,#3433,#3434,#3435,#3436,#3437,
#3438,#3439,#3440,#3441,#3442,#3443,#3444,#3445,#3446,#3447,#3448,#3449,
#3450,#3451));
#3704=AXIS2_PLACEMENT_3D('',#5358,#4339,#4340);
#3705=AXIS2_PLACEMENT_3D('',#5359,#4341,#4342);
#3706=AXIS2_PLACEMENT_3D('',#5363,#4344,#4345);
#3707=AXIS2_PLACEMENT_3D('',#5364,#4346,#4347);
#3708=AXIS2_PLACEMENT_3D('',#5367,#4348,#4349);
#3709=AXIS2_PLACEMENT_3D('',#5369,#4350,#4351);
#3710=AXIS2_PLACEMENT_3D('',#5370,#4352,#4353);
#3711=AXIS2_PLACEMENT_3D('',#5373,#4355,#4356);
#3712=AXIS2_PLACEMENT_3D('',#5374,#4357,#4358);
#3713=AXIS2_PLACEMENT_3D('',#5375,#4359,#4360);
#3714=AXIS2_PLACEMENT_3D('',#5377,#4361,#4362);
#3715=AXIS2_PLACEMENT_3D('',#5381,#4364,#4365);
#3716=AXIS2_PLACEMENT_3D('',#5383,#4366,#4367);
#3717=AXIS2_PLACEMENT_3D('',#5384,#4368,#4369);
#3718=AXIS2_PLACEMENT_3D('',#5385,#4370,#4371);
#3719=AXIS2_PLACEMENT_3D('',#5395,#4377,#4378);
#3720=AXIS2_PLACEMENT_3D('',#5405,#4384,#4385);
#3721=AXIS2_PLACEMENT_3D('',#5407,#4386,#4387);
#3722=AXIS2_PLACEMENT_3D('',#5410,#4389,#4390);
#3723=AXIS2_PLACEMENT_3D('',#5411,#4391,#4392);
#3724=AXIS2_PLACEMENT_3D('',#5413,#4393,#4394);
#3725=AXIS2_PLACEMENT_3D('',#5416,#4396,#4397);
#3726=AXIS2_PLACEMENT_3D('',#5417,#4398,#4399);
#3727=AXIS2_PLACEMENT_3D('',#5418,#4400,#4401);
#3728=AXIS2_PLACEMENT_3D('',#5420,#4402,#4403);
#3729=AXIS2_PLACEMENT_3D('',#5423,#4405,#4406);
#3730=AXIS2_PLACEMENT_3D('',#5424,#4407,#4408);
#3731=AXIS2_PLACEMENT_3D('',#5425,#4409,#4410);
#3732=AXIS2_PLACEMENT_3D('',#5434,#4415,#4416);
#3733=AXIS2_PLACEMENT_3D('',#5436,#4417,#4418);
#3734=AXIS2_PLACEMENT_3D('',#5440,#4420,#4421);
#3735=AXIS2_PLACEMENT_3D('',#5442,#4423,#4424);
#3736=AXIS2_PLACEMENT_3D('',#5445,#4425,#4426);
#3737=AXIS2_PLACEMENT_3D('',#5449,#4428,#4429);
#3738=AXIS2_PLACEMENT_3D('',#5451,#4431,#4432);
#3739=AXIS2_PLACEMENT_3D('',#5457,#4436,#4437);
#3740=AXIS2_PLACEMENT_3D('',#5459,#4438,#4439);
#3741=AXIS2_PLACEMENT_3D('',#5462,#4441,#4442);
#3742=AXIS2_PLACEMENT_3D('',#5463,#4443,#4444);
#3743=AXIS2_PLACEMENT_3D('',#5464,#4445,#4446);
#3744=AXIS2_PLACEMENT_3D('',#5473,#4451,#4452);
#3745=AXIS2_PLACEMENT_3D('',#5482,#4457,#4458);
#3746=AXIS2_PLACEMENT_3D('',#5492,#4464,#4465);
#3747=AXIS2_PLACEMENT_3D('',#5502,#4471,#4472);
#3748=AXIS2_PLACEMENT_3D('',#5505,#4473,#4474);
#3749=AXIS2_PLACEMENT_3D('',#5509,#4476,#4477);
#3750=AXIS2_PLACEMENT_3D('',#5511,#4478,#4479);
#3751=AXIS2_PLACEMENT_3D('',#5513,#4481,#4482);
#3752=AXIS2_PLACEMENT_3D('',#5516,#4483,#4484);
#3753=AXIS2_PLACEMENT_3D('',#5520,#4486,#4487);
#3754=AXIS2_PLACEMENT_3D('',#5522,#4489,#4490);
#3755=AXIS2_PLACEMENT_3D('',#5528,#4494,#4495);
#3756=AXIS2_PLACEMENT_3D('',#5530,#4496,#4497);
#3757=AXIS2_PLACEMENT_3D('',#5533,#4499,#4500);
#3758=AXIS2_PLACEMENT_3D('',#5534,#4501,#4502);
#3759=AXIS2_PLACEMENT_3D('',#5536,#4503,#4504);
#3760=AXIS2_PLACEMENT_3D('',#5539,#4506,#4507);
#3761=AXIS2_PLACEMENT_3D('',#5540,#4508,#4509);
#3762=AXIS2_PLACEMENT_3D('',#5546,#4513,#4514);
#3763=AXIS2_PLACEMENT_3D('',#5548,#4515,#4516);
#3764=AXIS2_PLACEMENT_3D('',#5551,#4518,#4519);
#3765=AXIS2_PLACEMENT_3D('',#5552,#4520,#4521);
#3766=AXIS2_PLACEMENT_3D('',#5567,#4532,#4533);
#3767=AXIS2_PLACEMENT_3D('',#5569,#4534,#4535);
#3768=AXIS2_PLACEMENT_3D('',#5571,#4537,#4538);
#3769=AXIS2_PLACEMENT_3D('',#5581,#4545,#4546);
#3770=AXIS2_PLACEMENT_3D('',#5585,#4549,#4550);
#3771=AXIS2_PLACEMENT_3D('',#5587,#4552,#4553);
#3772=AXIS2_PLACEMENT_3D('',#5593,#4557,#4558);
#3773=AXIS2_PLACEMENT_3D('',#5603,#4564,#4565);
#3774=AXIS2_PLACEMENT_3D('',#5605,#4567,#4568);
#3775=AXIS2_PLACEMENT_3D('',#5613,#4573,#4574);
#3776=AXIS2_PLACEMENT_3D('',#5616,#4577,#4578);
#3777=AXIS2_PLACEMENT_3D('',#5618,#4580,#4581);
#3778=AXIS2_PLACEMENT_3D('',#5619,#4582,#4583);
#3779=AXIS2_PLACEMENT_3D('',#5620,#4584,#4585);
#3780=AXIS2_PLACEMENT_3D('',#5621,#4586,#4587);
#3781=AXIS2_PLACEMENT_3D('',#5622,#4588,#4589);
#3782=AXIS2_PLACEMENT_3D('',#5623,#4590,#4591);
#3783=AXIS2_PLACEMENT_3D('',#5628,#4596,#4597);
#3784=AXIS2_PLACEMENT_3D('',#5630,#4599,#4600);
#3785=AXIS2_PLACEMENT_3D('',#5632,#4602,#4603);
#3786=AXIS2_PLACEMENT_3D('',#5634,#4605,#4606);
#3787=AXIS2_PLACEMENT_3D('',#5635,#4607,#4608);
#3788=AXIS2_PLACEMENT_3D('',#5637,#4610,#4611);
#3789=AXIS2_PLACEMENT_3D('',#5638,#4612,#4613);
#3790=AXIS2_PLACEMENT_3D('',#5651,#4620,#4621);
#3791=AXIS2_PLACEMENT_3D('',#5664,#4628,#4629);
#3792=AXIS2_PLACEMENT_3D('',#5672,#4634,#4635);
#3793=AXIS2_PLACEMENT_3D('',#5674,#4636,#4637);
#3794=AXIS2_PLACEMENT_3D('',#5675,#4638,#4639);
#3795=AXIS2_PLACEMENT_3D('',#5678,#4641,#4642);
#3796=AXIS2_PLACEMENT_3D('',#5679,#4643,#4644);
#3797=AXIS2_PLACEMENT_3D('',#5689,#4650,#4651);
#3798=AXIS2_PLACEMENT_3D('',#5698,#4656,#4657);
#3799=AXIS2_PLACEMENT_3D('',#5699,#4658,#4659);
#3800=AXIS2_PLACEMENT_3D('',#5700,#4660,#4661);
#3801=AXIS2_PLACEMENT_3D('',#5701,#4662,#4663);
#3802=AXIS2_PLACEMENT_3D('',#5703,#4664,#4665);
#3803=AXIS2_PLACEMENT_3D('',#5704,#4666,#4667);
#3804=AXIS2_PLACEMENT_3D('',#5706,#4669,#4670);
#3805=AXIS2_PLACEMENT_3D('',#5712,#4674,#4675);
#3806=AXIS2_PLACEMENT_3D('',#5718,#4679,#4680);
#3807=AXIS2_PLACEMENT_3D('',#5722,#4683,#4684);
#3808=AXIS2_PLACEMENT_3D('',#5728,#4688,#4689);
#3809=AXIS2_PLACEMENT_3D('',#5732,#4692,#4693);
#3810=AXIS2_PLACEMENT_3D('',#5736,#4695,#4696);
#3811=AXIS2_PLACEMENT_3D('',#5741,#4699,#4700);
#3812=AXIS2_PLACEMENT_3D('',#5745,#4702,#4703);
#3813=AXIS2_PLACEMENT_3D('',#5749,#4705,#4706);
#3814=AXIS2_PLACEMENT_3D('',#5756,#4710,#4711);
#3815=AXIS2_PLACEMENT_3D('',#5759,#4713,#4714);
#3816=AXIS2_PLACEMENT_3D('',#5760,#4715,#4716);
#3817=AXIS2_PLACEMENT_3D('',#5764,#4719,#4720);
#3818=AXIS2_PLACEMENT_3D('',#5772,#4724,#4725);
#3819=AXIS2_PLACEMENT_3D('',#5776,#4728,#4729);
#3820=AXIS2_PLACEMENT_3D('',#5780,#4732,#4733);
#3821=AXIS2_PLACEMENT_3D('',#5782,#4734,#4735);
#3822=AXIS2_PLACEMENT_3D('',#5784,#4737,#4738);
#3823=AXIS2_PLACEMENT_3D('',#5788,#4740,#4741);
#3824=AXIS2_PLACEMENT_3D('',#5792,#4743,#4744);
#3825=AXIS2_PLACEMENT_3D('',#5795,#4746,#4747);
#3826=AXIS2_PLACEMENT_3D('',#5799,#4749,#4750);
#3827=AXIS2_PLACEMENT_3D('',#5802,#4752,#4753);
#3828=AXIS2_PLACEMENT_3D('',#5803,#4754,#4755);
#3829=AXIS2_PLACEMENT_3D('',#5805,#4757,#4758);
#3830=AXIS2_PLACEMENT_3D('',#5807,#4760,#4761);
#3831=AXIS2_PLACEMENT_3D('',#5809,#4763,#4764);
#3832=AXIS2_PLACEMENT_3D('',#5812,#4767,#4768);
#3833=AXIS2_PLACEMENT_3D('',#5814,#4770,#4771);
#3834=AXIS2_PLACEMENT_3D('',#5816,#4773,#4774);
#3835=AXIS2_PLACEMENT_3D('',#5817,#4775,#4776);
#3836=AXIS2_PLACEMENT_3D('',#5819,#4778,#4779);
#3837=AXIS2_PLACEMENT_3D('',#5821,#4781,#4782);
#3838=AXIS2_PLACEMENT_3D('',#5823,#4784,#4785);
#3839=AXIS2_PLACEMENT_3D('',#5825,#4787,#4788);
#3840=AXIS2_PLACEMENT_3D('',#5829,#4791,#4792);
#3841=AXIS2_PLACEMENT_3D('',#5830,#4793,#4794);
#4339=DIRECTION('axis',(0.,0.,1.));
#4340=DIRECTION('refdir',(1.,0.,0.));
#4341=DIRECTION('center_axis',(-2.44876222201709E-16,0.0208291764396898,
0.999783049170591));
#4342=DIRECTION('ref_axis',(1.,-7.39048179408127E-33,2.44929359829471E-16));
#4343=DIRECTION('',(1.,2.87786876793731E-15,1.84972715848191E-16));
#4344=DIRECTION('center_axis',(-2.44876222201709E-16,0.0208291764396898,
0.999783049170591));
#4345=DIRECTION('ref_axis',(1.,-7.39048179408127E-33,2.44929359829471E-16));
#4346=DIRECTION('center_axis',(2.44876222201709E-16,-0.0208291764396898,
-0.999783049170591));
#4347=DIRECTION('ref_axis',(1.,-7.39048179408127E-33,2.44929359829471E-16));
#4348=DIRECTION('center_axis',(1.22464679914735E-16,0.,-1.));
#4349=DIRECTION('ref_axis',(0.,-1.,0.));
#4350=DIRECTION('center_axis',(1.7319121124633E-16,0.707104673835204,-0.707108888531611));
#4351=DIRECTION('ref_axis',(1.73190695094883E-16,-0.707108888531611,-0.707104673835204));
#4352=DIRECTION('center_axis',(1.22464679914735E-16,0.,-1.));
#4353=DIRECTION('ref_axis',(0.,-1.,0.));
#4354=DIRECTION('',(2.44876222201709E-16,-0.0208291764396898,-0.999783049170591));
#4355=DIRECTION('center_axis',(-1.24988949526429E-16,-0.0208291764396907,
0.999783049170591));
#4356=DIRECTION('ref_axis',(5.10167685114853E-18,-0.999783049170591,-0.0208291764396907));
#4357=DIRECTION('center_axis',(-1.24988949526429E-16,-0.0208291764396907,
0.999783049170591));
#4358=DIRECTION('ref_axis',(5.10167685114853E-18,-0.999783049170591,-0.0208291764396907));
#4359=DIRECTION('center_axis',(2.44876222201709E-16,-0.0208291764396898,
-0.999783049170591));
#4360=DIRECTION('ref_axis',(1.,-7.39048179408127E-33,2.44929359829471E-16));
#4361=DIRECTION('center_axis',(1.1988727267528E-16,-0.0208291764396907,
-0.999783049170591));
#4362=DIRECTION('ref_axis',(1.,-2.60341688269759E-18,1.19967526759308E-16));
#4363=DIRECTION('',(2.44876222201709E-16,-0.0208291764396898,-0.999783049170591));
#4364=DIRECTION('center_axis',(-1.22464679914735E-16,0.,1.));
#4365=DIRECTION('ref_axis',(0.,-1.,0.));
#4366=DIRECTION('center_axis',(-5.16151446417155E-22,0.707104673835204,
0.707108888531611));
#4367=DIRECTION('ref_axis',(-1.73190695094883E-16,-0.707108888531611,0.707104673835204));
#4368=DIRECTION('center_axis',(-1.22464679914735E-16,0.,1.));
#4369=DIRECTION('ref_axis',(0.,-1.,0.));
#4370=DIRECTION('center_axis',(1.22464679914735E-16,0.,-1.));
#4371=DIRECTION('ref_axis',(-1.22464679914735E-16,-1.,-1.49975978266185E-32));
#4372=DIRECTION('',(-1.,1.22464679914735E-16,-1.22464679914735E-16));
#4373=DIRECTION('',(1.22464679914735E-16,1.,1.49975978266186E-32));
#4374=DIRECTION('',(1.,-1.22464679914735E-16,1.22464679914735E-16));
#4375=DIRECTION('',(-1.22464679914735E-16,-1.,-1.49975978266186E-32));
#4376=DIRECTION('',(-1.,1.22464679914735E-16,-1.22464679914735E-16));
#4377=DIRECTION('center_axis',(-1.22464679914735E-16,0.,1.));
#4378=DIRECTION('ref_axis',(1.22464679914735E-16,1.,1.49975978266185E-32));
#4379=DIRECTION('',(-1.,1.22464679914735E-16,-1.22464679914735E-16));
#4380=DIRECTION('',(1.22464679914735E-16,1.,1.49975978266186E-32));
#4381=DIRECTION('',(-1.,1.22464679914735E-16,-1.22464679914735E-16));
#4382=DIRECTION('',(-1.22464679914735E-16,-1.,-1.49975978266186E-32));
#4383=DIRECTION('',(-1.,1.22464679914735E-16,-1.22464679914735E-16));
#4384=DIRECTION('center_axis',(0.,0.0208291764396898,-0.999783049170591));
#4385=DIRECTION('ref_axis',(1.,0.,0.));
#4386=DIRECTION('center_axis',(1.22464679914735E-16,0.,-1.));
#4387=DIRECTION('ref_axis',(0.,-1.,0.));
#4388=DIRECTION('',(0.,0.0208291764396898,-0.999783049170591));
#4389=DIRECTION('center_axis',(-1.22464679914735E-16,0.,1.));
#4390=DIRECTION('ref_axis',(0.,-1.,0.));
#4391=DIRECTION('center_axis',(0.,-1.,0.));
#4392=DIRECTION('ref_axis',(-1.,0.,0.));
#4393=DIRECTION('center_axis',(-1.22464679914735E-16,-1.,-1.49975978266186E-32));
#4394=DIRECTION('ref_axis',(1.,-1.22464679914735E-16,1.22464679914735E-16));
#4395=DIRECTION('',(0.,-1.,0.));
#4396=DIRECTION('center_axis',(1.83667601732677E-48,-1.,2.73691106313441E-48));
#4397=DIRECTION('ref_axis',(-1.,-1.83667601732677E-48,0.));
#4398=DIRECTION('center_axis',(-1.83667601732677E-48,1.,-2.73691106313441E-48));
#4399=DIRECTION('ref_axis',(-1.,-1.83667601732677E-48,0.));
#4400=DIRECTION('center_axis',(0.,-1.,0.));
#4401=DIRECTION('ref_axis',(-1.,0.,0.));
#4402=DIRECTION('center_axis',(-1.22464679914735E-16,-1.,-1.49975978266186E-32));
#4403=DIRECTION('ref_axis',(1.,-1.22464679914735E-16,1.22464679914735E-16));
#4404=DIRECTION('',(0.,-1.,0.));
#4405=DIRECTION('center_axis',(1.83667601732677E-48,-1.,2.24927940568994E-64));
#4406=DIRECTION('ref_axis',(-1.,-1.83667601732677E-48,0.));
#4407=DIRECTION('center_axis',(-1.83667601732677E-48,1.,-2.24927940568994E-64));
#4408=DIRECTION('ref_axis',(-1.,-1.83667601732677E-48,0.));
#4409=DIRECTION('center_axis',(1.,-1.22464679914735E-16,1.22464679914735E-16));
#4410=DIRECTION('ref_axis',(1.22464679914735E-16,0.,-1.));
#4411=DIRECTION('',(-1.22464679914735E-16,0.,1.));
#4412=DIRECTION('',(1.22464679914735E-16,1.,1.49975978266186E-32));
#4413=DIRECTION('',(1.22464679914735E-16,0.,-1.));
#4414=DIRECTION('',(1.22464679914735E-16,1.,1.49975978266186E-32));
#4415=DIRECTION('center_axis',(1.22464679914735E-16,1.,1.49975978266186E-32));
#4416=DIRECTION('ref_axis',(1.22464679914735E-16,1.0252425757274E-46,-1.));
#4417=DIRECTION('center_axis',(-1.22464679914735E-16,-1.,-1.49975978266186E-32));
#4418=DIRECTION('ref_axis',(1.22464679914735E-16,1.0252425757274E-46,-1.));
#4419=DIRECTION('',(1.22464679914735E-16,1.,1.49975978266186E-32));
#4420=DIRECTION('center_axis',(1.22464679914735E-16,1.,1.49975978266186E-32));
#4421=DIRECTION('ref_axis',(1.22464679914735E-16,1.0252425757274E-46,-1.));
#4422=DIRECTION('',(1.22464679914735E-16,1.,1.49975978266186E-32));
#4423=DIRECTION('center_axis',(1.22464679914735E-16,1.,1.49975978266186E-32));
#4424=DIRECTION('ref_axis',(1.22464679914735E-16,1.0252425757274E-46,-1.));
#4425=DIRECTION('center_axis',(1.22464679914735E-16,1.,1.49975978266186E-32));
#4426=DIRECTION('ref_axis',(1.22464679914735E-16,1.0252425757274E-46,-1.));
#4427=DIRECTION('',(1.22464679914735E-16,1.,1.49975978266186E-32));
#4428=DIRECTION('center_axis',(-1.22464679914735E-16,-1.,-1.49975978266186E-32));
#4429=DIRECTION('ref_axis',(1.22464679914735E-16,1.0252425757274E-46,-1.));
#4430=DIRECTION('',(1.22464679914735E-16,1.,1.49975978266186E-32));
#4431=DIRECTION('center_axis',(-1.,1.22464679914735E-16,-1.22464679914735E-16));
#4432=DIRECTION('ref_axis',(-1.22464679914735E-16,0.,1.));
#4433=DIRECTION('',(1.22464679914735E-16,0.,-1.));
#4434=DIRECTION('',(1.22464679914735E-16,1.,1.49975978266186E-32));
#4435=DIRECTION('',(-1.22464679914735E-16,0.,1.));
#4436=DIRECTION('center_axis',(1.22464679914735E-16,1.,1.49975978266186E-32));
#4437=DIRECTION('ref_axis',(1.,-1.22464679914735E-16,1.22464679914735E-16));
#4438=DIRECTION('center_axis',(1.22464679914735E-16,1.,1.49975978266186E-32));
#4439=DIRECTION('ref_axis',(1.,-1.22464679914735E-16,1.22464679914735E-16));
#4440=DIRECTION('',(1.22464679914735E-16,1.,1.49975978266186E-32));
#4441=DIRECTION('center_axis',(-1.22464679914735E-16,-1.,-1.49975978266186E-32));
#4442=DIRECTION('ref_axis',(1.,-1.22464679914735E-16,1.22464679914735E-16));
#4443=DIRECTION('center_axis',(-1.22464679914735E-16,-1.,-1.49975978266186E-32));
#4444=DIRECTION('ref_axis',(1.,-1.22464679914735E-16,1.22464679914735E-16));
#4445=DIRECTION('center_axis',(1.,-1.22464679914735E-16,1.22464679914735E-16));
#4446=DIRECTION('ref_axis',(-1.22464679914735E-16,0.,1.));
#4447=DIRECTION('',(-1.22464679914735E-16,0.,1.));
#4448=DIRECTION('',(-1.22464679914735E-16,-1.,-1.49975978266186E-32));
#4449=DIRECTION('',(-1.22464679914735E-16,0.,1.));
#4450=DIRECTION('',(-1.22464679914735E-16,-1.,-1.49975978266186E-32));
#4451=DIRECTION('center_axis',(1.,-1.22464679914735E-16,1.22464679914735E-16));
#4452=DIRECTION('ref_axis',(-1.22464679914735E-16,0.,1.));
#4453=DIRECTION('',(-1.22464679914735E-16,0.,1.));
#4454=DIRECTION('',(1.22464679914735E-16,1.,1.49975978266186E-32));
#4455=DIRECTION('',(-1.22464679914735E-16,0.,1.));
#4456=DIRECTION('',(-1.22464679914735E-16,-1.,-1.49975978266186E-32));
#4457=DIRECTION('center_axis',(1.,-1.22464679914735E-16,1.22464679914735E-16));
#4458=DIRECTION('ref_axis',(-1.22464679914735E-16,0.,1.));
#4459=DIRECTION('',(-1.22464679914735E-16,0.,1.));
#4460=DIRECTION('',(-1.7319121124633E-16,-0.707108888531611,0.707104673835204));
#4461=DIRECTION('',(-5.16151446417155E-22,-0.707108888531611,-0.707104673835204));
#4462=DIRECTION('',(-1.22464679914735E-16,0.,1.));
#4463=DIRECTION('',(1.1988727267528E-16,0.999783049170591,0.0208291764396907));
#4464=DIRECTION('center_axis',(1.,-1.22464679914735E-16,1.22464679914735E-16));
#4465=DIRECTION('ref_axis',(-1.22464679914735E-16,0.,1.));
#4466=DIRECTION('',(-1.22464679914735E-16,0.,1.));
#4467=DIRECTION('',(-1.24988949526429E-16,-0.999783049170591,0.0208291764396907));
#4468=DIRECTION('',(-1.22464679914735E-16,0.,1.));
#4469=DIRECTION('',(1.7319121124633E-16,0.707108888531611,-0.707104673835204));
#4470=DIRECTION('',(5.16151446417155E-22,0.707108888531611,0.707104673835204));
#4471=DIRECTION('center_axis',(1.22464679914735E-16,1.,1.49975978266186E-32));
#4472=DIRECTION('ref_axis',(-0.70710688994201,8.6595618942252E-17,0.707106672431068));
#4473=DIRECTION('center_axis',(-1.22464679914735E-16,-1.,-1.49975978266186E-32));
#4474=DIRECTION('ref_axis',(-0.70710688994201,8.6595618942252E-17,0.707106672431068));
#4475=DIRECTION('',(1.22464679914735E-16,1.,1.49975978266186E-32));
#4476=DIRECTION('center_axis',(1.22464679914735E-16,1.,1.49975978266186E-32));
#4477=DIRECTION('ref_axis',(-0.70710688994201,8.6595618942252E-17,0.707106672431068));
#4478=DIRECTION('center_axis',(1.22464679914735E-16,1.,1.49975978266186E-32));
#4479=DIRECTION('ref_axis',(-0.70710688994201,8.6595618942252E-17,0.707106672431068));
#4480=DIRECTION('',(1.22464679914735E-16,1.,1.49975978266186E-32));
#4481=DIRECTION('center_axis',(1.22464679914735E-16,1.,1.49975978266186E-32));
#4482=DIRECTION('ref_axis',(-0.382683511888619,4.68652137920864E-17,-0.923879499571558));
#4483=DIRECTION('center_axis',(-1.22464679914735E-16,-1.,-1.49975978266186E-32));
#4484=DIRECTION('ref_axis',(-0.70710688994201,8.6595618942252E-17,0.707106672431068));
#4485=DIRECTION('',(1.22464679914735E-16,1.,1.49975978266186E-32));
#4486=DIRECTION('center_axis',(-1.22464679914735E-16,-1.,-1.49975978266186E-32));
#4487=DIRECTION('ref_axis',(-0.70710688994201,8.6595618942252E-17,0.707106672431068));
#4488=DIRECTION('',(1.22464679914735E-16,1.,1.49975978266186E-32));
#4489=DIRECTION('center_axis',(-1.,1.22464679914735E-16,-1.22464679914735E-16));
#4490=DIRECTION('ref_axis',(-1.22464679914735E-16,0.,1.));
#4491=DIRECTION('',(-1.22464679914735E-16,0.,1.));
#4492=DIRECTION('',(1.22464679914735E-16,1.,1.49975978266186E-32));
#4493=DIRECTION('',(-1.22464679914735E-16,0.,1.));
#4494=DIRECTION('center_axis',(1.22464679914735E-16,1.,1.49975978266186E-32));
#4495=DIRECTION('ref_axis',(-0.619814087082361,7.5905333781185E-17,0.784748684264115));
#4496=DIRECTION('center_axis',(-1.22464679914735E-16,-1.,-1.49975978266186E-32));
#4497=DIRECTION('ref_axis',(-0.619814087082361,7.5905333781185E-17,0.784748684264115));
#4498=DIRECTION('',(1.22464679914735E-16,1.,1.49975978266186E-32));
#4499=DIRECTION('center_axis',(1.22464679914735E-16,1.,1.49975978266186E-32));
#4500=DIRECTION('ref_axis',(-0.619814087082361,7.5905333781185E-17,0.784748684264115));
#4501=DIRECTION('center_axis',(1.22464679914735E-16,1.,1.49975978266186E-32));
#4502=DIRECTION('ref_axis',(0.149925588670012,-1.83605892275013E-17,0.988697283227758));
#4503=DIRECTION('center_axis',(1.22464679914735E-16,1.,1.49975978266186E-32));
#4504=DIRECTION('ref_axis',(0.149925588670012,-1.83605892275013E-17,0.988697283227758));
#4505=DIRECTION('',(1.22464679914735E-16,1.,1.49975978266186E-32));
#4506=DIRECTION('center_axis',(-1.22464679914735E-16,-1.,-1.49975978266186E-32));
#4507=DIRECTION('ref_axis',(0.149925588670012,-1.83605892275013E-17,0.988697283227758));
#4508=DIRECTION('center_axis',(0.999999975140088,-1.22464676870274E-16,
-0.000222979425718486));
#4509=DIRECTION('ref_axis',(-0.000222979425718486,2.73071039982008E-20,
-0.999999975140088));
#4510=DIRECTION('',(0.000222979425718486,-2.73071039982008E-20,0.999999975140088));
#4511=DIRECTION('',(1.22464679914735E-16,1.,1.49975978266186E-32));
#4512=DIRECTION('',(-0.000222979425718486,2.73071039982008E-20,-0.999999975140088));
#4513=DIRECTION('center_axis',(1.22464679914735E-16,1.,1.49975978266186E-32));
#4514=DIRECTION('ref_axis',(-0.999999975140088,1.22464676870274E-16,0.000222979425690885));
#4515=DIRECTION('center_axis',(1.22464679914735E-16,1.,1.49975978266186E-32));
#4516=DIRECTION('ref_axis',(-0.999999975140088,1.22464676870274E-16,0.000222979425690885));
#4517=DIRECTION('',(1.22464679914735E-16,1.,1.49975978266186E-32));
#4518=DIRECTION('center_axis',(-1.22464679914735E-16,-1.,-1.49975978266186E-32));
#4519=DIRECTION('ref_axis',(-0.999999975140088,1.22464676870274E-16,0.000222979425690885));
#4520=DIRECTION('center_axis',(-2.84598478402269E-15,3.33535017790927E-31,
1.));
#4521=DIRECTION('ref_axis',(1.,-1.22464679914735E-16,2.84598478402269E-15));
#4522=DIRECTION('',(-1.,1.22464679914735E-16,-2.84598478402269E-15));
#4523=DIRECTION('',(-1.,1.22464679914735E-16,-2.84598478402269E-15));
#4524=DIRECTION('',(1.22464679914735E-16,1.,1.49975978266186E-32));
#4525=DIRECTION('',(1.,-1.22464679914735E-16,2.75774059927426E-15));
#4526=DIRECTION('',(1.22464679914735E-16,1.,1.49975978266186E-32));
#4527=DIRECTION('',(-1.,1.22464679914735E-16,-2.75774059927426E-15));
#4528=DIRECTION('',(-1.,1.22464679914735E-16,-2.84598478402269E-15));
#4529=DIRECTION('',(-1.,1.22464679914735E-16,-2.75774059927426E-15));
#4530=DIRECTION('',(1.,-1.22464679914735E-16,2.75774059927426E-15));
#4531=DIRECTION('',(-1.,1.22464679914735E-16,-2.84598478402269E-15));
#4532=DIRECTION('center_axis',(1.22464679914735E-16,1.,1.49975978266186E-32));
#4533=DIRECTION('ref_axis',(-0.707106824182888,8.65956108890821E-17,0.707106738190205));
#4534=DIRECTION('center_axis',(1.22464679914735E-16,1.,1.49975978266186E-32));
#4535=DIRECTION('ref_axis',(-0.707106824182888,8.65956108890821E-17,0.707106738190205));
#4536=DIRECTION('',(1.22464679914735E-16,1.,1.49975978266186E-32));
#4537=DIRECTION('center_axis',(-1.22464679914735E-16,-1.,-1.49975978266186E-32));
#4538=DIRECTION('ref_axis',(1.,-1.22464679914735E-16,1.22464679914735E-16));
#4539=DIRECTION('',(-1.,1.22464679914735E-16,-1.22464679914735E-16));
#4540=DIRECTION('',(1.22464679914735E-16,0.,-1.));
#4541=DIRECTION('',(-1.,1.22464679914735E-16,-2.68280906625521E-15));
#4542=DIRECTION('',(1.22464679914735E-16,0.,-1.));
#4543=DIRECTION('',(1.,-1.22464679914735E-16,1.22464679914735E-16));
#4544=DIRECTION('',(-1.,1.22464679914735E-16,-2.68280906625521E-15));
#4545=DIRECTION('center_axis',(-1.,1.22464679914735E-16,-1.22464679914735E-16));
#4546=DIRECTION('ref_axis',(1.22464679914735E-16,0.,-1.));
#4547=DIRECTION('',(1.22464679914735E-16,0.,-1.));
#4548=DIRECTION('',(-1.22464679914735E-16,-1.,-1.49975978266186E-32));
#4549=DIRECTION('center_axis',(1.22464679914735E-16,0.,-1.));
#4550=DIRECTION('ref_axis',(1.,-1.22464679914735E-16,1.22464679914735E-16));
#4551=DIRECTION('',(1.,-1.22464679914735E-16,1.22464679914735E-16));
#4552=DIRECTION('center_axis',(-1.,1.22464679914735E-16,-1.22464679914735E-16));
#4553=DIRECTION('ref_axis',(1.22464679914735E-16,0.,-1.));
#4554=DIRECTION('',(-1.22464679914735E-16,-1.,-1.49975978266186E-32));
#4555=DIRECTION('',(1.22464679914735E-16,0.,-1.));
#4556=DIRECTION('',(-1.22464679914735E-16,-1.,-1.49975978266186E-32));
#4557=DIRECTION('center_axis',(-1.,1.22464679914735E-16,-1.22464679914735E-16));
#4558=DIRECTION('ref_axis',(1.22464679914735E-16,0.,-1.));
#4559=DIRECTION('',(1.22464679914735E-16,0.,-1.));
#4560=DIRECTION('',(-1.1988727267528E-16,-0.999783049170591,-0.0208291764396907));
#4561=DIRECTION('',(1.22464679914735E-16,0.,-1.));
#4562=DIRECTION('',(5.16151446417155E-22,0.707108888531611,0.707104673835204));
#4563=DIRECTION('',(1.7319121124633E-16,0.707108888531611,-0.707104673835204));
#4564=DIRECTION('center_axis',(-1.22464679914735E-16,-1.,-1.49975978266186E-32));
#4565=DIRECTION('ref_axis',(1.22464679914735E-16,1.0252425757274E-46,-1.));
#4566=DIRECTION('',(1.22464679914735E-16,0.,-1.));
#4567=DIRECTION('center_axis',(-1.,1.22464679914735E-16,-1.22464679914735E-16));
#4568=DIRECTION('ref_axis',(1.22464679914735E-16,0.,-1.));
#4569=DIRECTION('',(1.22464679914735E-16,0.,-1.));
#4570=DIRECTION('',(-5.16151446417155E-22,-0.707108888531611,-0.707104673835204));
#4571=DIRECTION('',(-1.7319121124633E-16,-0.707108888531611,0.707104673835204));
#4572=DIRECTION('',(1.24988949526429E-16,0.999783049170591,-0.0208291764396907));
#4573=DIRECTION('center_axis',(1.22464679914735E-16,1.,1.49975978266186E-32));
#4574=DIRECTION('ref_axis',(1.22464679914735E-16,1.0252425757274E-46,-1.));
#4575=DIRECTION('',(-1.,1.22464679914735E-16,-1.22464679914735E-16));
#4576=DIRECTION('',(1.,-1.22464679914735E-16,1.22464679914735E-16));
#4577=DIRECTION('center_axis',(1.7319121124633E-16,0.707104673835204,-0.707108888531611));
#4578=DIRECTION('ref_axis',(-5.16151446399029E-22,-0.707108888531611,-0.707104673835204));
#4579=DIRECTION('',(-1.,1.22464679914735E-16,-1.22464679914735E-16));
#4580=DIRECTION('center_axis',(5.16151446417155E-22,-0.707104673835204,
-0.707108888531611));
#4581=DIRECTION('ref_axis',(-1.7319121124633E-16,-0.707108888531611,0.707104673835204));
#4582=DIRECTION('center_axis',(-1.1988727267528E-16,0.0208291764396907,
0.999783049170591));
#4583=DIRECTION('ref_axis',(1.24988949526429E-16,0.999783049170591,-0.0208291764396907));
#4584=DIRECTION('center_axis',(1.22464679914735E-16,1.,1.49975978266186E-32));
#4585=DIRECTION('ref_axis',(0.192330993613606,-2.35537535705732E-17,0.981330112090525));
#4586=DIRECTION('center_axis',(1.22464679914735E-16,1.,1.49975978266186E-32));
#4587=DIRECTION('ref_axis',(0.192330993613606,-2.35537535705732E-17,0.981330112090525));
#4588=DIRECTION('center_axis',(-1.22464679914735E-16,-1.,-1.49975978266186E-32));
#4589=DIRECTION('ref_axis',(0.192330993613606,-2.35537535705732E-17,0.981330112090525));
#4590=DIRECTION('center_axis',(1.22464679914735E-16,0.,-1.));
#4591=DIRECTION('ref_axis',(-1.,1.22464679914735E-16,-1.22464679914735E-16));
#4592=DIRECTION('',(-1.,1.22464679914735E-16,-1.22464679914735E-16));
#4593=DIRECTION('',(1.,-1.22464679914735E-16,1.22464679914735E-16));
#4594=DIRECTION('',(1.,-1.22464679914735E-16,1.22464679914735E-16));
#4595=DIRECTION('',(1.,-1.22464679914735E-16,1.22464679914735E-16));
#4596=DIRECTION('center_axis',(1.24988949526429E-16,0.0208291764396907,
-0.999783049170591));
#4597=DIRECTION('ref_axis',(-1.1988727267528E-16,-0.999783049170591,-0.0208291764396907));
#4598=DIRECTION('',(-1.,1.22464679914735E-16,-1.22464679914735E-16));
#4599=DIRECTION('center_axis',(1.22464679914735E-16,1.,1.49975978266186E-32));
#4600=DIRECTION('ref_axis',(1.22464679914735E-16,1.0252425757274E-46,-1.));
#4601=DIRECTION('',(1.,-1.22464679914735E-16,1.22464679914735E-16));
#4602=DIRECTION('center_axis',(-5.16151446417155E-22,0.707104673835204,
0.707108888531611));
#4603=DIRECTION('ref_axis',(1.7319121124633E-16,0.707108888531611,-0.707104673835204));
#4604=DIRECTION('',(-1.,1.22464679914735E-16,-1.22464679914735E-16));
#4605=DIRECTION('center_axis',(-1.7319121124633E-16,-0.707104673835204,
0.707108888531611));
#4606=DIRECTION('ref_axis',(5.16151446399029E-22,0.707108888531611,0.707104673835204));
#4607=DIRECTION('center_axis',(-1.22464679914735E-16,-1.,-1.49975978266186E-32));
#4608=DIRECTION('ref_axis',(1.22464679914735E-16,1.0252425757274E-46,-1.));
#4609=DIRECTION('',(-1.,1.22464679914735E-16,-1.22464679914735E-16));
#4610=DIRECTION('center_axis',(-1.22464679914735E-16,0.,1.));
#4611=DIRECTION('ref_axis',(-1.,1.22464679914735E-16,-1.22464679914735E-16));
#4612=DIRECTION('center_axis',(-1.,1.22464679914735E-16,-1.22464679914735E-16));
#4613=DIRECTION('ref_axis',(-1.22464679914735E-16,0.,1.));
#4614=DIRECTION('',(1.22464679914735E-16,0.,-1.));
#4615=DIRECTION('',(1.22464679914735E-16,1.,1.49975978266186E-32));
#4616=DIRECTION('',(1.7319121124633E-16,0.707108888531611,-0.707104673835204));
#4617=DIRECTION('',(1.22464679914735E-16,1.,0.));
#4618=DIRECTION('',(0.,-1.49975978266186E-32,1.));
#4619=DIRECTION('',(-1.22464679914735E-16,-1.,-1.49975978266186E-32));
#4620=DIRECTION('center_axis',(-1.,1.22464679914735E-16,-1.22464679914735E-16));
#4621=DIRECTION('ref_axis',(-1.22464679914735E-16,0.,1.));
#4622=DIRECTION('',(1.22464679914735E-16,0.,-1.));
#4623=DIRECTION('',(1.22464679914735E-16,1.,1.49975978266186E-32));
#4624=DIRECTION('',(0.,-1.49975978266186E-32,1.));
#4625=DIRECTION('',(-1.22464679914735E-16,-1.,0.));
#4626=DIRECTION('',(-6.28038757050967E-15,-0.707108888531611,-0.707104673835204));
#4627=DIRECTION('',(1.22464679914735E-16,1.,1.49975978266186E-32));
#4628=DIRECTION('center_axis',(-1.22464679914735E-16,0.,1.));
#4629=DIRECTION('ref_axis',(1.,-1.22464679914735E-16,1.22464679914735E-16));
#4630=DIRECTION('',(1.,-1.22464679914735E-16,2.77139240997905E-15));
#4631=DIRECTION('',(1.22464679914735E-16,1.,1.49975978266186E-32));
#4632=DIRECTION('',(1.22464679914735E-16,1.,1.49975978266186E-32));
#4633=DIRECTION('',(1.,-1.22464679914735E-16,1.22464679914735E-16));
#4634=DIRECTION('center_axis',(-1.22464679914735E-16,-1.,-1.49975978266186E-32));
#4635=DIRECTION('ref_axis',(1.,-1.22464679914735E-16,1.22464679914735E-16));
#4636=DIRECTION('center_axis',(1.22464679914735E-16,1.,1.49975978266186E-32));
#4637=DIRECTION('ref_axis',(1.,-1.22464679914735E-16,1.22464679914735E-16));
#4638=DIRECTION('center_axis',(1.22464679914735E-16,1.,1.49975978266186E-32));
#4639=DIRECTION('ref_axis',(1.,-1.22464679914735E-16,1.22464679914735E-16));
#4640=DIRECTION('',(1.22464679914735E-16,1.,1.49975978266186E-32));
#4641=DIRECTION('center_axis',(-1.22464679914735E-16,-1.,-1.49975978266186E-32));
#4642=DIRECTION('ref_axis',(1.,-1.22464679914735E-16,1.22464679914735E-16));
#4643=DIRECTION('center_axis',(2.76087478076931E-15,-3.23112048484961E-31,
-1.));
#4644=DIRECTION('ref_axis',(-1.,1.22464679914735E-16,-2.76087478076931E-15));
#4645=DIRECTION('',(1.,-1.22464679914735E-16,2.76087478076931E-15));
#4646=DIRECTION('',(1.22464679914735E-16,1.,1.49975978266186E-32));
#4647=DIRECTION('',(1.,-1.22464679914735E-16,4.87374585786276E-17));
#4648=DIRECTION('',(1.22464679914735E-16,1.,1.49975978266186E-32));
#4649=DIRECTION('',(-1.,1.22464679914735E-16,-4.87374585786276E-17));
#4650=DIRECTION('center_axis',(1.,-1.22464679914735E-16,1.22464679914735E-16));
#4651=DIRECTION('ref_axis',(1.22464679914735E-16,0.,-1.));
#4652=DIRECTION('',(-1.22464679914735E-16,0.,1.));
#4653=DIRECTION('',(1.22464679914735E-16,1.,1.49975978266186E-32));
#4654=DIRECTION('',(1.22464679914735E-16,0.,-1.));
#4655=DIRECTION('',(1.22464679914735E-16,1.,1.49975978266186E-32));
#4656=DIRECTION('center_axis',(1.22464679914735E-16,1.,1.49975978266186E-32));
#4657=DIRECTION('ref_axis',(-1.89882151931499E-15,2.17540971751502E-31,
1.));
#4658=DIRECTION('center_axis',(1.22464679914735E-16,1.,1.49975978266186E-32));
#4659=DIRECTION('ref_axis',(-1.89882151931499E-15,2.17540971751502E-31,
1.));
#4660=DIRECTION('center_axis',(-1.22464679914735E-16,-1.,-1.49975978266186E-32));
#4661=DIRECTION('ref_axis',(-1.89882151931499E-15,2.17540971751502E-31,
1.));
#4662=DIRECTION('center_axis',(1.22464679914735E-16,1.,1.49975978266186E-32));
#4663=DIRECTION('ref_axis',(-2.12086612424002E-15,2.4473359322044E-31,1.));
#4664=DIRECTION('center_axis',(-1.22464679914735E-16,-1.,-1.49975978266186E-32));
#4665=DIRECTION('ref_axis',(-2.12086612424002E-15,2.4473359322044E-31,1.));
#4666=DIRECTION('center_axis',(1.22464679914735E-16,1.,1.49975978266186E-32));
#4667=DIRECTION('ref_axis',(-2.12086612424002E-15,2.4473359322044E-31,1.));
#4668=DIRECTION('',(1.22464679914735E-16,1.,1.49975978266186E-32));
#4669=DIRECTION('center_axis',(-1.,1.22464679914735E-16,-1.22464679914735E-16));
#4670=DIRECTION('ref_axis',(-1.22464679914735E-16,0.,1.));
#4671=DIRECTION('',(-1.22464679914735E-16,0.,1.));
#4672=DIRECTION('',(-1.22464679914735E-16,0.,1.));
#4673=DIRECTION('',(1.22464679914735E-16,1.,1.49975978266186E-32));
#4674=DIRECTION('center_axis',(0.,0.,-1.));
#4675=DIRECTION('ref_axis',(-1.22464679914735E-16,-1.,0.));
#4676=DIRECTION('',(-1.,1.22464679914735E-16,0.));
#4677=DIRECTION('',(1.22464679914735E-16,1.,0.));
#4678=DIRECTION('',(1.,0.,0.));
#4679=DIRECTION('center_axis',(0.,0.707104673835204,-0.707108888531611));
#4680=DIRECTION('ref_axis',(-6.28038757050967E-15,-0.707108888531611,-0.707104673835204));
#4681=DIRECTION('',(6.28038757050967E-15,0.707108888531611,0.707104673835204));
#4682=DIRECTION('',(1.,1.22465409865287E-16,1.22464679914735E-16));
#4683=DIRECTION('center_axis',(0.,0.707104673835204,0.707108888531611));
#4684=DIRECTION('ref_axis',(1.7319121124633E-16,0.707108888531611,-0.707104673835204));
#4685=DIRECTION('',(-1.,1.22465409865287E-16,-1.22464679914735E-16));
#4686=DIRECTION('',(-1.7319121124633E-16,-0.707108888531611,0.707104673835204));
#4687=DIRECTION('',(-1.,0.,0.));
#4688=DIRECTION('center_axis',(0.,0.,1.));
#4689=DIRECTION('ref_axis',(1.22464679914735E-16,1.,0.));
#4690=DIRECTION('',(-1.22464679914735E-16,-1.,0.));
#4691=DIRECTION('',(1.,-1.22464679914735E-16,0.));
#4692=DIRECTION('center_axis',(-1.22464679914735E-16,-1.,-1.49975978266186E-32));
#4693=DIRECTION('ref_axis',(1.,-1.22464679914735E-16,1.22464679914735E-16));
#4694=DIRECTION('',(0.707106606671929,-8.65955842516724E-17,0.707106955701123));
#4695=DIRECTION('center_axis',(-1.22464679914735E-16,-1.,-1.49975978266186E-32));
#4696=DIRECTION('ref_axis',(0.707106824182887,-8.65956108890821E-17,-0.707106738190205));
#4697=DIRECTION('',(1.,-1.22464679914735E-16,1.22464679914735E-16));
#4698=DIRECTION('',(0.,1.49975978266186E-32,-1.));
#4699=DIRECTION('center_axis',(-1.22464679914735E-16,-1.,-1.49975978266186E-32));
#4700=DIRECTION('ref_axis',(-0.192330993613605,2.35537535705731E-17,-0.981330112090526));
#4701=DIRECTION('',(0.797940776019378,-9.77195617261287E-17,0.602735860859127));
#4702=DIRECTION('center_axis',(-1.22464679914735E-16,-1.,-1.49975978266186E-32));
#4703=DIRECTION('ref_axis',(0.619814087082361,-7.5905333781185E-17,-0.784748684264115));
#4704=DIRECTION('',(1.22464679914735E-16,0.,-1.));
#4705=DIRECTION('center_axis',(-1.22464679914735E-16,-1.,-1.49975978266186E-32));
#4706=DIRECTION('ref_axis',(0.70710688994201,-8.6595618942252E-17,-0.707106672431068));
#4707=DIRECTION('',(0.707106672431068,-8.65955923048443E-17,0.707106889942011));
#4708=DIRECTION('',(1.22464679914735E-16,0.,-1.));
#4709=DIRECTION('',(1.,-1.22464679914735E-16,2.76087478076931E-15));
#4710=DIRECTION('center_axis',(1.22464679914735E-16,1.,1.49975978266186E-32));
#4711=DIRECTION('ref_axis',(0.999999975140088,-1.22464676870274E-16,-0.000222979425697547));
#4712=DIRECTION('',(-0.000222979425718486,2.73071039982009E-20,-0.999999975140088));
#4713=DIRECTION('center_axis',(1.22464679914735E-16,1.,1.49975978266186E-32));
#4714=DIRECTION('ref_axis',(-0.149925588670012,1.83605892275013E-17,-0.988697283227758));
#4715=DIRECTION('center_axis',(-1.22464679914735E-16,0.,1.));
#4716=DIRECTION('ref_axis',(1.,-1.22464679914735E-16,1.22464679914735E-16));
#4717=DIRECTION('',(-1.,1.22464679914735E-16,-1.22464679914735E-16));
#4718=DIRECTION('',(1.22464679914735E-16,1.,1.49975978266186E-32));
#4719=DIRECTION('center_axis',(-1.22464679914735E-16,-1.,-1.49975978266186E-32));
#4720=DIRECTION('ref_axis',(1.,-1.22464679914735E-16,1.22464679914735E-16));
#4721=DIRECTION('',(1.,-1.22464679914735E-16,1.22464679914735E-16));
#4722=DIRECTION('',(-1.22464679914735E-16,0.,1.));
#4723=DIRECTION('',(1.,-1.22464679914735E-16,2.77139240997905E-15));
#4724=DIRECTION('center_axis',(1.22464679914735E-16,1.,1.49975978266186E-32));
#4725=DIRECTION('ref_axis',(0.707106824182887,-8.65956108890821E-17,-0.707106738190205));
#4726=DIRECTION('',(-1.,1.22464679914735E-16,-4.87374585786276E-17));
#4727=DIRECTION('',(-1.22464679914735E-16,0.,1.));
#4728=DIRECTION('center_axis',(0.707106955701123,-8.6595626995421E-17,-0.707106606671929));
#4729=DIRECTION('ref_axis',(-0.707106606671929,8.65955842516724E-17,-0.707106955701123));
#4730=DIRECTION('',(-0.707106606671929,8.65955842516724E-17,-0.707106955701123));
#4731=DIRECTION('',(1.22464679914735E-16,1.,1.49975978266186E-32));
#4732=DIRECTION('center_axis',(1.22464679914735E-16,1.,1.49975978266186E-32));
#4733=DIRECTION('ref_axis',(-0.192330993613605,2.35537535705731E-17,-0.981330112090526));
#4734=DIRECTION('center_axis',(1.22464679914735E-16,1.,1.49975978266186E-32));
#4735=DIRECTION('ref_axis',(-0.192330993613605,2.35537535705731E-17,-0.981330112090526));
#4736=DIRECTION('',(1.22464679914735E-16,1.,1.49975978266186E-32));
#4737=DIRECTION('center_axis',(-1.22464679914735E-16,-1.,-1.49975978266186E-32));
#4738=DIRECTION('ref_axis',(1.,-1.22464679914735E-16,1.22464679914735E-16));
#4739=DIRECTION('',(0.707106672431068,-8.65955923048443E-17,0.707106889942011));
#4740=DIRECTION('center_axis',(-1.22464679914735E-16,-1.,-1.49975978266186E-32));
#4741=DIRECTION('ref_axis',(0.70710688994201,-8.6595618942252E-17,-0.707106672431068));
#4742=DIRECTION('',(1.22464679914735E-16,0.,-1.));
#4743=DIRECTION('center_axis',(1.22464679914735E-16,1.,1.49975978266186E-32));
#4744=DIRECTION('ref_axis',(0.619814087082361,-7.5905333781185E-17,-0.784748684264115));
#4745=DIRECTION('',(-0.797940776019378,9.77195617261287E-17,-0.602735860859127));
#4746=DIRECTION('center_axis',(-1.22464679914735E-16,-1.,-1.49975978266186E-32));
#4747=DIRECTION('ref_axis',(-0.149925588670012,1.83605892275013E-17,-0.988697283227758));
#4748=DIRECTION('',(0.000222979425718486,-2.73071039982009E-20,0.999999975140088));
#4749=DIRECTION('center_axis',(-1.22464679914735E-16,-1.,-1.49975978266186E-32));
#4750=DIRECTION('ref_axis',(0.999999975140088,-1.22464676870274E-16,-0.000222979425697547));
#4751=DIRECTION('',(1.,-1.22464679914735E-16,4.87374585786276E-17));
#4752=DIRECTION('center_axis',(1.22464679914735E-16,1.,1.49975978266186E-32));
#4753=DIRECTION('ref_axis',(0.707106824182887,-8.65956108890821E-17,-0.707106738190205));
#4754=DIRECTION('center_axis',(1.,-1.22464679914735E-16,1.22464679914735E-16));
#4755=DIRECTION('ref_axis',(1.22464679914735E-16,0.,-1.));
#4756=DIRECTION('',(1.22464679914735E-16,1.,1.49975978266186E-32));
#4757=DIRECTION('center_axis',(1.22464679914735E-16,0.,-1.));
#4758=DIRECTION('ref_axis',(-1.,1.22464679914735E-16,-1.22464679914735E-16));
#4759=DIRECTION('',(1.22464679914735E-16,1.,1.49975978266186E-32));
#4760=DIRECTION('center_axis',(1.,-1.22464679914735E-16,1.22464679914735E-16));
#4761=DIRECTION('ref_axis',(1.22464679914735E-16,0.,-1.));
#4762=DIRECTION('',(-1.22464679914735E-16,-1.,-1.49975978266186E-32));
#4763=DIRECTION('center_axis',(2.76087478076931E-15,-3.23112048484961E-31,
-1.));
#4764=DIRECTION('ref_axis',(-1.,1.22464679914735E-16,-2.76087478076931E-15));
#4765=DIRECTION('',(1.22464679914735E-16,1.,1.49975978266186E-32));
#4766=DIRECTION('',(1.22464679914735E-16,1.,1.49975978266186E-32));
#4767=DIRECTION('center_axis',(1.22464679914735E-16,1.,1.49975978266186E-32));
#4768=DIRECTION('ref_axis',(0.999999975140088,-1.22464676870274E-16,-0.000222979425697547));
#4769=DIRECTION('',(1.22464679914735E-16,1.,1.49975978266186E-32));
#4770=DIRECTION('center_axis',(-0.999999975140088,1.22464676870274E-16,
0.000222979425718486));
#4771=DIRECTION('ref_axis',(0.000222979425718486,-2.73071039982009E-20,
0.999999975140088));
#4772=DIRECTION('',(1.22464679914735E-16,1.,1.49975978266186E-32));
#4773=DIRECTION('center_axis',(1.22464679914735E-16,1.,1.49975978266186E-32));
#4774=DIRECTION('ref_axis',(-0.149925588670012,1.83605892275013E-17,-0.988697283227758));
#4775=DIRECTION('center_axis',(0.602735860859127,-7.38138542732454E-17,
-0.797940776019378));
#4776=DIRECTION('ref_axis',(-0.797940776019378,9.77195617261287E-17,-0.602735860859127));
#4777=DIRECTION('',(1.22464679914735E-16,1.,1.49975978266186E-32));
#4778=DIRECTION('center_axis',(1.22464679914735E-16,1.,1.49975978266186E-32));
#4779=DIRECTION('ref_axis',(0.619814087082361,-7.5905333781185E-17,-0.784748684264115));
#4780=DIRECTION('',(1.22464679914735E-16,1.,1.49975978266186E-32));
#4781=DIRECTION('center_axis',(1.,-1.22464679914735E-16,1.22464679914735E-16));
#4782=DIRECTION('ref_axis',(1.22464679914735E-16,0.,-1.));
#4783=DIRECTION('',(1.22464679914735E-16,1.,1.49975978266186E-32));
#4784=DIRECTION('center_axis',(1.22464679914735E-16,1.,1.49975978266186E-32));
#4785=DIRECTION('ref_axis',(0.382683511888619,-4.68652137920864E-17,0.923879499571558));
#4786=DIRECTION('',(-1.22464679914735E-16,-1.,-1.49975978266186E-32));
#4787=DIRECTION('center_axis',(-1.22464679914735E-16,0.,1.));
#4788=DIRECTION('ref_axis',(1.,-1.22464679914735E-16,1.22464679914735E-16));
#4789=DIRECTION('',(1.22464679914735E-16,1.,1.49975978266186E-32));
#4790=DIRECTION('',(1.22464679914735E-16,1.,1.49975978266186E-32));
#4791=DIRECTION('center_axis',(1.22464679914735E-16,1.,1.49975978266186E-32));
#4792=DIRECTION('ref_axis',(0.707106824182887,-8.65956108890821E-17,-0.707106738190205));
#4793=DIRECTION('center_axis',(-0.707106889942011,8.65956189422523E-17,
0.707106672431068));
#4794=DIRECTION('ref_axis',(0.707106672431068,-8.65955923048443E-17,0.707106889942011));
#5358=CARTESIAN_POINT('',(0.,0.,0.));
#5359=CARTESIAN_POINT('Origin',(55.4902124404907,-4.00000013411045,0.145828066207017));
#5360=CARTESIAN_POINT('',(54.1678121566157,-5.5000937214608,0.177080560468535));
#5361=CARTESIAN_POINT('',(56.8126127243658,-5.5000937214608,0.177080560468536));
#5362=CARTESIAN_POINT('',(55.4902111948072,-5.5000937214608,0.177080560468535));
#5363=CARTESIAN_POINT('Origin',(55.4902124404907,-4.00000013411045,0.145828066207017));
#5364=CARTESIAN_POINT('Origin',(55.4902124404907,-4.00000013411045,0.145828066207017));
#5365=CARTESIAN_POINT('',(55.7596018087023,-2.00000023841859,0.999999909568344));
#5366=CARTESIAN_POINT('',(53.4902124404907,-3.98220457731446,0.999999909568344));
#5367=CARTESIAN_POINT('Origin',(55.4902124404907,-3.98220457731446,0.999999909568344));
#5368=CARTESIAN_POINT('',(55.2208230722792,-2.00000023841859,0.999999909568344));
#5369=CARTESIAN_POINT('Origin',(55.4902124404907,-4.02437963145607,-1.02436741723056));
#5370=CARTESIAN_POINT('Origin',(55.4902124404907,-3.98220457731446,0.999999909568344));
#5371=CARTESIAN_POINT('',(53.4902124404907,-3.99869735870019,0.208360196357335));
#5372=CARTESIAN_POINT('',(53.4902124404907,-4.00000013411045,0.145828066207016));
#5373=CARTESIAN_POINT('Origin',(55.4902124404907,-3.9986973587002,0.208360196357335));
#5374=CARTESIAN_POINT('Origin',(55.4902124404907,-3.9986973587002,0.208360196357335));
#5375=CARTESIAN_POINT('Origin',(55.4902124404907,-4.00000013411045,0.145828066207017));
#5376=CARTESIAN_POINT('',(53.4902124404907,-3.90325229314834,4.78964351987318));
#5377=CARTESIAN_POINT('Origin',(55.4902124404907,-3.90325229314834,4.78964351987318));
#5378=CARTESIAN_POINT('',(53.4902124404907,-3.91970364728078,3.99999228017381));
#5379=CARTESIAN_POINT('',(53.4902124404907,-4.00000013411045,0.145828066207016));
#5380=CARTESIAN_POINT('',(54.9277733864728,-2.00000023841859,3.99999228017381));
#5381=CARTESIAN_POINT('Origin',(55.4902124404907,-3.91970364728078,3.99999228017381));
#5382=CARTESIAN_POINT('',(56.0526514945086,-2.00000023841859,3.99999228017381));
#5383=CARTESIAN_POINT('Origin',(55.4902124404907,-3.88052558675829,5.88050641971165));
#5384=CARTESIAN_POINT('Origin',(55.4902124404907,-3.91970364728078,3.99999228017381));
#5385=CARTESIAN_POINT('Origin',(55.4902099491237,-2.00000023841859,3.99999228017381));
#5386=CARTESIAN_POINT('',(59.4902099491237,-2.00000023841859,3.99999228017381));
#5387=CARTESIAN_POINT('',(55.4902099491237,-2.00000023841859,3.99999228017381));
#5388=CARTESIAN_POINT('',(59.4902099491237,-13.9999999994186,3.99999228017381));
#5389=CARTESIAN_POINT('',(59.4902099491237,-2.00000023841859,3.99999228017381));
#5390=CARTESIAN_POINT('',(51.4902099491237,-13.9999999994186,3.99999228017381));
#5391=CARTESIAN_POINT('',(55.4902099491237,-14.,3.99999228017381));
#5392=CARTESIAN_POINT('',(51.4902099491237,-2.00000023841859,3.99999228017381));
#5393=CARTESIAN_POINT('',(51.4902099491237,-2.00000023841859,3.99999228017381));
#5394=CARTESIAN_POINT('',(55.4902099491237,-2.00000023841859,3.99999228017381));
#5395=CARTESIAN_POINT('Origin',(55.4902099491237,-13.9999999701977,0.999999909568344));
#5396=CARTESIAN_POINT('',(51.4902099491237,-2.00000023841859,0.999999909568344));
#5397=CARTESIAN_POINT('',(55.4902099491237,-2.00000023841859,0.999999909568344));
#5398=CARTESIAN_POINT('',(51.4902099491237,-13.9999999994186,0.999999909568344));
#5399=CARTESIAN_POINT('',(51.4902099491237,-2.00000023841859,0.999999909568344));
#5400=CARTESIAN_POINT('',(59.4902099491237,-13.9999999994186,0.999999909568344));
#5401=CARTESIAN_POINT('',(55.4902099491237,-14.,0.999999909568344));
#5402=CARTESIAN_POINT('',(59.4902099491237,-2.00000023841859,0.999999909568344));
#5403=CARTESIAN_POINT('',(59.4902099491237,-2.00000023841859,0.999999909568344));
#5404=CARTESIAN_POINT('',(55.4902099491237,-2.00000023841859,0.999999909568344));
#5405=CARTESIAN_POINT('Origin',(55.4902124404907,-12.0000001341105,105.854167938232));
#5406=CARTESIAN_POINT('',(53.4902124404907,-11.9780379165298,104.799999861885));
#5407=CARTESIAN_POINT('Origin',(55.4902124404907,-11.9780379165298,104.799999861885));
#5408=CARTESIAN_POINT('',(53.4902124404907,-11.9213427352736,102.078678577114));
#5409=CARTESIAN_POINT('',(53.4902124404907,-12.0000001341105,105.854167938232));
#5410=CARTESIAN_POINT('Origin',(55.4902124404907,-11.9213427352736,102.078678577114));
#5411=CARTESIAN_POINT('Origin',(10.0000020566038,-4.00000000000001,2.50000086324266));
#5412=CARTESIAN_POINT('',(11.500002191775,-8.,2.50000086324266));
#5413=CARTESIAN_POINT('Origin',(10.0000020566037,-8.,2.50000086324266));
#5414=CARTESIAN_POINT('',(11.500002191775,-12.,2.50000086324266));
#5415=CARTESIAN_POINT('',(11.500002191775,-4.00000000000001,2.50000086324266));
#5416=CARTESIAN_POINT('Origin',(10.0000020566038,-12.,2.50000086324266));
#5417=CARTESIAN_POINT('Origin',(10.0000020566038,-12.,2.50000086324266));
#5418=CARTESIAN_POINT('Origin',(100.979994297411,-4.00000000000001,103.500004749034));
#5419=CARTESIAN_POINT('',(102.479993922177,-8.00000000000001,103.500004749034));
#5420=CARTESIAN_POINT('Origin',(100.979994297411,-8.00000000000001,103.500004749034));
#5421=CARTESIAN_POINT('',(102.479993922177,-12.,103.500004749034));
#5422=CARTESIAN_POINT('',(102.479993922178,-4.00000000000001,103.500004749034));
#5423=CARTESIAN_POINT('Origin',(100.979994297411,-12.,103.500004749034));
#5424=CARTESIAN_POINT('Origin',(100.979994297411,-12.,103.500004749034));
#5425=CARTESIAN_POINT('Origin',(110.980422389614,-16.,44.959851174522));
#5426=CARTESIAN_POINT('',(110.980422389614,-16.,4.9999960948711));
#5427=CARTESIAN_POINT('',(110.980422389614,-16.,44.959851174522));
#5428=CARTESIAN_POINT('',(110.980422389614,-16.,4.9999960948711));
#5429=CARTESIAN_POINT('',(110.980422389614,-9.00000000000001,4.9999960948711));
#5430=CARTESIAN_POINT('',(110.980422389614,-16.,4.9999960948711));
#5431=CARTESIAN_POINT('',(110.980422389614,-9.00000000000001,44.959851174522));
#5432=CARTESIAN_POINT('',(110.980422389614,-9.00000000000001,4.9999960948711));
#5433=CARTESIAN_POINT('',(110.980422389614,-16.,44.959851174522));
#5434=CARTESIAN_POINT('Origin',(105.980422389614,-16.,4.99999609487108));
#5435=CARTESIAN_POINT('',(105.980422389614,-16.,-3.90512892134431E-6));
#5436=CARTESIAN_POINT('Origin',(105.980422389614,-16.,4.99999609487108));
#5437=CARTESIAN_POINT('',(105.980422389614,-8.00000000000001,-3.90512892134431E-6));
#5438=CARTESIAN_POINT('',(105.980422389614,-16.,-3.90512892134431E-6));
#5439=CARTESIAN_POINT('',(110.980422389614,-8.00000000000001,4.99999609487108));
#5440=CARTESIAN_POINT('Origin',(105.980422389614,-8.00000000000001,4.99999609487108));
#5441=CARTESIAN_POINT('',(110.980422389614,-16.,4.99999609487108));
#5442=CARTESIAN_POINT('Origin',(100.980422389614,-16.,9.99999609487106));
#5443=CARTESIAN_POINT('',(105.980422389614,-16.,9.99999609487106));
#5444=CARTESIAN_POINT('',(100.980422389614,-16.,4.99999609487106));
#5445=CARTESIAN_POINT('Origin',(100.980422389614,-16.,9.99999609487106));
#5446=CARTESIAN_POINT('',(105.980422389614,-9.00000000000001,9.99999609487106));
#5447=CARTESIAN_POINT('',(105.980422389614,-16.,9.99999609487106));
#5448=CARTESIAN_POINT('',(100.980422389614,-9.00000000000001,4.99999609487106));
#5449=CARTESIAN_POINT('Origin',(100.980422389614,-9.00000000000001,9.99999609487106));
#5450=CARTESIAN_POINT('',(100.980422389614,-16.,4.99999609487106));
#5451=CARTESIAN_POINT('Origin',(105.980422389614,-16.,9.99999609487106));
#5452=CARTESIAN_POINT('',(105.980422389614,-16.,40.7547899280026));
#5453=CARTESIAN_POINT('',(105.980422389614,-16.,9.99999609487106));
#5454=CARTESIAN_POINT('',(105.980422389614,-9.00000000000001,40.7547899280026));
#5455=CARTESIAN_POINT('',(105.980422389614,-16.,40.7547899280026));
#5456=CARTESIAN_POINT('',(105.980422389614,-9.00000000000001,9.99999609487106));
#5457=CARTESIAN_POINT('Origin',(100.97999641745,-16.,2.50000986180084));
#5458=CARTESIAN_POINT('',(99.2299941278536,-13.2,2.50000986180084));
#5459=CARTESIAN_POINT('Origin',(100.97999641745,-13.2,2.50000986180084));
#5460=CARTESIAN_POINT('',(99.2299941278536,-8.00000000000001,2.50000986180084));
#5461=CARTESIAN_POINT('',(99.2299941278536,-16.,2.50000986180084));
#5462=CARTESIAN_POINT('Origin',(100.97999641745,-8.00000000000001,2.50000986180084));
#5463=CARTESIAN_POINT('Origin',(100.97999641745,-13.2,2.50000986180084));
#5464=CARTESIAN_POINT('Origin',(60.4902099491237,-8.00000000000001,3.49999037282518));
#5465=CARTESIAN_POINT('',(60.4902099491237,-8.00000000000001,3.49999037282518));
#5466=CARTESIAN_POINT('',(60.4902099491237,-8.00000000000001,4.99999609487094));
#5467=CARTESIAN_POINT('',(60.4902099491237,-8.00000000000001,2.99999323384806));
#5468=CARTESIAN_POINT('',(60.4902099491237,-14.,3.49999037282518));
#5469=CARTESIAN_POINT('',(60.4902099491237,-8.00000000000001,3.49999037282518));
#5470=CARTESIAN_POINT('',(60.4902099491237,-14.,4.99999609487094));
#5471=CARTESIAN_POINT('',(60.4902099491237,-14.,-1.45337795352698));
#5472=CARTESIAN_POINT('',(60.4902099491237,-12.,4.99999609487094));
#5473=CARTESIAN_POINT('Origin',(60.4902099491237,-8.00000000000001,-3.90512906345286E-6));
#5474=CARTESIAN_POINT('',(60.4902099491237,-8.00000000000001,-3.90512906345286E-6));
#5475=CARTESIAN_POINT('',(60.4902099491237,-8.00000000000001,1.50000181691698));
#5476=CARTESIAN_POINT('',(60.4902099491237,-8.00000000000001,1.24999609487094));
#5477=CARTESIAN_POINT('',(60.4902099491237,-14.,-3.90512906345286E-6));
#5478=CARTESIAN_POINT('',(60.4902099491237,-12.,-3.90512892134431E-6));
#5479=CARTESIAN_POINT('',(60.4902099491237,-14.,1.50000181691698));
#5480=CARTESIAN_POINT('',(60.4902099491237,-14.,-1.45337795352698));
#5481=CARTESIAN_POINT('',(60.4902099491237,-8.00000000000001,1.50000181691698));
#5482=CARTESIAN_POINT('Origin',(59.4902099491237,-6.99999986588956,0.999995141196762));
#5483=CARTESIAN_POINT('',(59.4902099491237,2.38418571552046E-7,0.291667847800766));
#5484=CARTESIAN_POINT('',(59.4902099491237,2.38418571552046E-7,0.999999909568344));
#5485=CARTESIAN_POINT('',(59.4902099491237,2.38418571552046E-7,0.999999909568344));
#5486=CARTESIAN_POINT('',(59.4902099491237,-1.00000000000001,1.99999418752245));
#5487=CARTESIAN_POINT('',(59.4902099491237,2.38418571552046E-7,0.999999909568344));
#5488=CARTESIAN_POINT('',(59.4902099491237,-1.00000000000001,1.99999418752245));
#5489=CARTESIAN_POINT('',(59.4902099491237,-13.9999999992512,-3.90533088293397E-6));
#5490=CARTESIAN_POINT('',(59.4902099491237,-14.,0.87499704854536));
#5491=CARTESIAN_POINT('',(59.4902099491237,2.38418571552046E-7,0.291667847800766));
#5492=CARTESIAN_POINT('Origin',(59.4902099491237,-6.99999986588956,3.99999704854539));
#5493=CARTESIAN_POINT('',(59.4902099491237,2.38418571552046E-7,3.99999228017381));
#5494=CARTESIAN_POINT('',(59.4902099491237,2.38418571552046E-7,4.70832434194139));
#5495=CARTESIAN_POINT('',(59.4902099491237,2.38418571552046E-7,4.70832434194139));
#5496=CARTESIAN_POINT('',(59.4902099491237,-13.9999999992512,4.99999609507296));
#5497=CARTESIAN_POINT('',(59.4902099491237,2.38418571552046E-7,4.70832434194139));
#5498=CARTESIAN_POINT('',(59.4902099491237,-14.,4.12499514119673));
#5499=CARTESIAN_POINT('',(59.4902099491237,-1.00000000000001,2.99999800221971));
#5500=CARTESIAN_POINT('',(59.4902099491237,-1.00000000000001,2.99999800221971));
#5501=CARTESIAN_POINT('',(59.4902099491237,2.38418571552046E-7,3.99999228017381));
#5502=CARTESIAN_POINT('Origin',(8.84895893454662,-16.,2.99999609487109));
#5503=CARTESIAN_POINT('',(6.72763826472058,-16.,5.1213161121643));
#5504=CARTESIAN_POINT('',(8.84895893454661,-16.,-3.90512892134431E-6));
#5505=CARTESIAN_POINT('Origin',(8.84895893454662,-16.,2.99999609487109));
#5506=CARTESIAN_POINT('',(6.72763826472058,-9.,5.1213161121643));
#5507=CARTESIAN_POINT('',(6.72763826472058,-16.,5.1213161121643));
#5508=CARTESIAN_POINT('',(6.61289924081467,-9.,4.99999646013235));
#5509=CARTESIAN_POINT('Origin',(8.84895893454662,-9.,2.99999609487109));
#5510=CARTESIAN_POINT('',(8.84896668275571,-9.,-3.90512567523723E-6));
#5511=CARTESIAN_POINT('Origin',(8.84895893454662,-9.,2.99999609487109));
#5512=CARTESIAN_POINT('',(8.84895893454661,-16.,-3.90512892134431E-6));
#5513=CARTESIAN_POINT('Origin',(23.7605935886074,-16.,14.7296319220772));
#5514=CARTESIAN_POINT('',(20.9321760059474,-16.,17.5580486346965));
#5515=CARTESIAN_POINT('',(27.7605794788478,-16.,14.7296306182628));
#5516=CARTESIAN_POINT('Origin',(23.7605935886074,-16.,14.7296319220772));
#5517=CARTESIAN_POINT('',(27.7605794788478,-9.,14.7296306182628));
#5518=CARTESIAN_POINT('',(27.7605794788478,-16.,14.7296306182628));
#5519=CARTESIAN_POINT('',(20.9321760059474,-9.,17.5580486346965));
#5520=CARTESIAN_POINT('Origin',(23.7605935886074,-9.,14.7296319220772));
#5521=CARTESIAN_POINT('',(20.9321760059474,-16.,17.5580486346965));
#5522=CARTESIAN_POINT('Origin',(27.7605794788478,-16.,14.7296306182628));
#5523=CARTESIAN_POINT('',(27.7605794788478,-16.,21.3985714008098));
#5524=CARTESIAN_POINT('',(27.7605794788478,-16.,14.7296306182628));
#5525=CARTESIAN_POINT('',(27.7605794788478,-9.,21.3985714008098));
#5526=CARTESIAN_POINT('',(27.7605794788478,-16.,21.3985714008098));
#5527=CARTESIAN_POINT('',(27.7605794788478,-9.,14.7296306182628));
#5528=CARTESIAN_POINT('Origin',(32.7605816884901,-16.,21.3985714008098));
#5529=CARTESIAN_POINT('',(29.6615098835109,-16.,25.3223165561443));
#5530=CARTESIAN_POINT('Origin',(32.7605816884901,-16.,21.3985714008098));
#5531=CARTESIAN_POINT('',(29.6615098835109,-9.,25.3223165561443));
#5532=CARTESIAN_POINT('',(29.6615098835109,-16.,25.3223165561443));
#5533=CARTESIAN_POINT('Origin',(32.7605816884901,-9.00000000000001,21.3985714008098));
#5534=CARTESIAN_POINT('Origin',(91.7027316808384,-16.,-53.4006783930403));
#5535=CARTESIAN_POINT('',(32.7605816882684,-16.,21.3985704065551));
#5536=CARTESIAN_POINT('Origin',(91.7027316808384,-16.,-53.4006783930403));
#5537=CARTESIAN_POINT('',(32.7605816882684,-9.00000000000001,21.3985704065551));
#5538=CARTESIAN_POINT('',(32.7605816882684,-16.,21.3985704065551));
#5539=CARTESIAN_POINT('Origin',(91.7027316808384,-9.00000000000001,-53.4006783930403));
#5540=CARTESIAN_POINT('Origin',(32.7605816882684,-16.,21.3985704065551));
#5541=CARTESIAN_POINT('',(32.7575942309482,-16.,8.00066503314802));
#5542=CARTESIAN_POINT('',(32.7605816884901,-16.,21.3985714008098));
#5543=CARTESIAN_POINT('',(32.7575942309482,-9.00000000000001,8.00066503314802));
#5544=CARTESIAN_POINT('',(32.7575942309482,-16.,8.00066503314802));
#5545=CARTESIAN_POINT('',(32.7605816884901,-9.00000000000001,21.3985714008098));
#5546=CARTESIAN_POINT('Origin',(35.7575941563685,-16.,7.99999609487094));
#5547=CARTESIAN_POINT('',(35.7575941563685,-16.,4.99999609487087));
#5548=CARTESIAN_POINT('Origin',(35.7575941563685,-16.,7.99999609487094));
#5549=CARTESIAN_POINT('',(35.7575941563685,-9.00000000000001,4.99999609487087));
#5550=CARTESIAN_POINT('',(35.7575941563685,-16.,4.99999609487087));
#5551=CARTESIAN_POINT('Origin',(35.7575941563685,-9.00000000000001,7.99999609487094));
#5552=CARTESIAN_POINT('Origin',(35.7575941563685,-16.,4.99999609487087));
#5553=CARTESIAN_POINT('',(51.4902099491237,-13.9999999992512,4.99999609507295));
#5554=CARTESIAN_POINT('',(45.6239020527461,-14.,4.9999960948709));
#5555=CARTESIAN_POINT('',(50.4902099491237,-14.,4.9999960948709));
#5556=CARTESIAN_POINT('',(45.6239020527461,-14.,4.9999960948709));
#5557=CARTESIAN_POINT('',(50.4902099491237,-8.00000000000001,4.9999960948709));
#5558=CARTESIAN_POINT('',(50.4902099491237,-12.,4.9999960948709));
#5559=CARTESIAN_POINT('',(6.61290645425235,-8.,4.99999609487078));
#5560=CARTESIAN_POINT('',(118.22869783717,-8.00000000000002,4.9999960948711));
#5561=CARTESIAN_POINT('',(6.61290645425235,-16.,4.99999609487078));
#5562=CARTESIAN_POINT('',(31.0515582016881,-9.,4.99999609487085));
#5563=CARTESIAN_POINT('',(100.980422389614,-16.,4.99999609487106));
#5564=CARTESIAN_POINT('',(31.0515582016881,-9.,4.99999609487085));
#5565=CARTESIAN_POINT('',(118.22869783717,-8.00000000000002,4.9999960948711));
#5566=CARTESIAN_POINT('',(45.6239020527461,-14.,4.9999960948709));
#5567=CARTESIAN_POINT('Origin',(8.84897443175212,-16.,2.99999609487078));
#5568=CARTESIAN_POINT('',(8.84897443175215,-8.,-3.90512918779784E-6));
#5569=CARTESIAN_POINT('Origin',(8.84897443175212,-8.,2.99999609487078));
#5570=CARTESIAN_POINT('',(8.84897443175215,-16.,-3.90512918779784E-6));
#5571=CARTESIAN_POINT('Origin',(58.4146984106833,-8.00000000000001,2.49999609487094));
#5572=CARTESIAN_POINT('',(50.4902099491237,-8.00000000000001,1.50000181691698));
#5573=CARTESIAN_POINT('',(59.4524541799035,-8.00000000000001,1.50000181691698));
#5574=CARTESIAN_POINT('',(50.4902099491237,-8.00000000000001,-3.90512908121643E-6));
#5575=CARTESIAN_POINT('',(50.4902099491237,-8.00000000000001,1.99999895589396));
#5576=CARTESIAN_POINT('',(105.980422389614,-8.00000000000001,-3.90512892134431E-6));
#5577=CARTESIAN_POINT('',(50.4902099491237,-8.00000000000001,3.49999037282518));
#5578=CARTESIAN_POINT('',(50.4902099491237,-8.00000000000001,3.74999609487092));
#5579=CARTESIAN_POINT('',(54.4524541799035,-8.00000000000001,3.49999037282518));
#5580=CARTESIAN_POINT('',(105.980422389614,-8.00000000000001,-3.90512892134431E-6));
#5581=CARTESIAN_POINT('Origin',(50.4902099491237,-8.00000000000001,4.9999960948709));
#5582=CARTESIAN_POINT('',(50.4902099491237,-14.,3.49999037282518));
#5583=CARTESIAN_POINT('',(50.4902099491237,-14.,6.66819775988521));
#5584=CARTESIAN_POINT('',(50.4902099491237,-8.00000000000001,3.49999037282518));
#5585=CARTESIAN_POINT('Origin',(50.4902099491237,-8.00000000000001,3.49999037282518));
#5586=CARTESIAN_POINT('',(50.4902099491237,-14.,3.49999037282518));
#5587=CARTESIAN_POINT('Origin',(50.4902099491237,-8.00000000000001,1.50000181691698));
#5588=CARTESIAN_POINT('',(50.4902099491237,-14.,1.50000181691698));
#5589=CARTESIAN_POINT('',(50.4902099491237,-8.00000000000001,1.50000181691698));
#5590=CARTESIAN_POINT('',(50.4902099491237,-14.,-3.90512908121643E-6));
#5591=CARTESIAN_POINT('',(50.4902099491237,-14.,6.66819775988521));
#5592=CARTESIAN_POINT('',(50.4902099491237,-12.,-3.90512892134431E-6));
#5593=CARTESIAN_POINT('Origin',(51.4902099491237,-6.99999986588956,0.999995141196762));
#5594=CARTESIAN_POINT('',(51.4902099491237,2.38418571552046E-7,0.999999909568344));
#5595=CARTESIAN_POINT('',(51.4902099491237,2.38418571552046E-7,0.291667847800766));
#5596=CARTESIAN_POINT('',(51.4902099491237,2.38418571552046E-7,0.999999909568344));
#5597=CARTESIAN_POINT('',(51.4902099491237,-13.9999999992512,-3.905330883632E-6));
#5598=CARTESIAN_POINT('',(51.4902099491237,2.38418571552046E-7,0.291667847800766));
#5599=CARTESIAN_POINT('',(51.4902099491237,-14.,0.87499704854536));
#5600=CARTESIAN_POINT('',(51.4902099491237,-1.00000000000001,1.99999418752245));
#5601=CARTESIAN_POINT('',(51.4902099491237,-1.00000000000001,1.99999418752245));
#5602=CARTESIAN_POINT('',(51.4902099491237,2.38418571552046E-7,0.999999909568344));
#5603=CARTESIAN_POINT('Origin',(55.4902099491237,-14.,4.24999323384806));
#5604=CARTESIAN_POINT('',(51.4902099491237,-14.,4.12499514119673));
#5605=CARTESIAN_POINT('Origin',(51.4902099491237,-6.99999986588956,3.99999704854539));
#5606=CARTESIAN_POINT('',(51.4902099491237,2.38418571552046E-7,4.70832434194139));
#5607=CARTESIAN_POINT('',(51.4902099491237,2.38418571552046E-7,3.99999228017381));
#5608=CARTESIAN_POINT('',(51.4902099491237,2.38418571552046E-7,4.70832434194139));
#5609=CARTESIAN_POINT('',(51.4902099491237,-1.00000000000001,2.99999800221971));
#5610=CARTESIAN_POINT('',(51.4902099491237,2.38418571552046E-7,3.99999228017381));
#5611=CARTESIAN_POINT('',(51.4902099491237,-1.00000000000001,2.99999800221971));
#5612=CARTESIAN_POINT('',(51.4902099491237,2.38418571552046E-7,4.70832434194139));
#5613=CARTESIAN_POINT('Origin',(55.4902099491237,2.38418571552046E-7,4.70832434194139));
#5614=CARTESIAN_POINT('',(55.4902099491237,2.38418571552046E-7,3.99999228017381));
#5615=CARTESIAN_POINT('',(55.4902099491237,2.38418571552046E-7,4.70832434194139));
#5616=CARTESIAN_POINT('Origin',(55.4902099491237,2.38418571552046E-7,3.99999228017381));
#5617=CARTESIAN_POINT('',(55.4902099491237,-1.00000000000001,2.99999800221971));
#5618=CARTESIAN_POINT('Origin',(55.4902099491237,-1.00000000000001,2.99999800221971));
#5619=CARTESIAN_POINT('Origin',(55.4902099491237,-13.9999999701977,4.99999609487108));
#5620=CARTESIAN_POINT('Origin',(91.7027316808383,-16.,-53.4006783930403));
#5621=CARTESIAN_POINT('Origin',(91.7027316808383,-9.00000000000001,-53.4006783930403));
#5622=CARTESIAN_POINT('Origin',(91.7027316808383,-16.,-53.4006783930403));
#5623=CARTESIAN_POINT('Origin',(105.980422389614,-16.,-3.90512890358075E-6));
#5624=CARTESIAN_POINT('',(110.980422389614,-16.,-3.90512890358075E-6));
#5625=CARTESIAN_POINT('',(80.7353161693691,-14.,-3.90512890358075E-6));
#5626=CARTESIAN_POINT('',(80.7353161693691,-14.,-3.90512890358075E-6));
#5627=CARTESIAN_POINT('',(80.7353161693691,-14.,-3.90512890358075E-6));
#5628=CARTESIAN_POINT('Origin',(55.4902099491237,2.38418571552046E-7,0.291667847800766));
#5629=CARTESIAN_POINT('',(55.4902099491237,2.38418571552046E-7,0.291667847800766));
#5630=CARTESIAN_POINT('Origin',(55.4902099491237,2.38418571552046E-7,0.999999909568344));
#5631=CARTESIAN_POINT('',(55.4902099491237,2.38418571552046E-7,0.999999909568344));
#5632=CARTESIAN_POINT('Origin',(55.4902099491237,-1.00000000000001,1.99999418752245));
#5633=CARTESIAN_POINT('',(55.4902099491237,-1.00000000000001,1.99999418752245));
#5634=CARTESIAN_POINT('Origin',(55.4902099491237,-2.00000023841859,0.999999909568344));
#5635=CARTESIAN_POINT('Origin',(55.4902099491237,-14.,0.749998955893957));
#5636=CARTESIAN_POINT('',(50.4902099491237,-14.,1.50000181691698));
#5637=CARTESIAN_POINT('Origin',(60.4902099491237,-8.00000000000001,1.50000181691698));
#5638=CARTESIAN_POINT('Origin',(50.4902099491237,-16.,100.999999909568));
#5639=CARTESIAN_POINT('',(50.4902099491237,-8.00000000000001,102.078678577114));
#5640=CARTESIAN_POINT('',(50.4902099491237,-8.00000000000001,100.999999909568));
#5641=CARTESIAN_POINT('',(50.4902099491237,-8.00000000000001,102.249999909568));
#5642=CARTESIAN_POINT('',(50.4902099491237,-14.0786711782186,102.078678577114));
#5643=CARTESIAN_POINT('',(50.4902099491237,-16.,102.078678577114));
#5644=CARTESIAN_POINT('',(50.4902099491237,-15.,103.000001907349));
#5645=CARTESIAN_POINT('',(50.4902099491237,-15.,103.000001907349));
#5646=CARTESIAN_POINT('',(50.4902099491237,-16.,103.000001907349));
#5647=CARTESIAN_POINT('',(50.4902099491237,-17.613291571013,103.000001907349));
#5648=CARTESIAN_POINT('',(50.4902099491237,-16.,100.999999909568));
#5649=CARTESIAN_POINT('',(50.4902099491237,-16.,77.7696691222254));
#5650=CARTESIAN_POINT('',(50.4902099491237,-16.,100.999999909568));
#5651=CARTESIAN_POINT('Origin',(50.4902099491237,-16.,104.799999861885));
#5652=CARTESIAN_POINT('',(50.4902099491237,-8.00000000000001,105.999999909569));
#5653=CARTESIAN_POINT('',(50.4902099491237,-8.00000000000001,104.799999861885));
#5654=CARTESIAN_POINT('',(50.4902099491237,-8.00000000000001,104.149999885727));
#5655=CARTESIAN_POINT('',(50.4902099491237,-16.,105.999999909569));
#5656=CARTESIAN_POINT('',(50.4902099491237,-16.,105.999999909568));
#5657=CARTESIAN_POINT('',(50.4902099491237,-16.,104.000005722046));
#5658=CARTESIAN_POINT('',(50.4902099491237,-16.,78.7000003970924));
#5659=CARTESIAN_POINT('',(50.4902099491237,-15.,104.000005722046));
#5660=CARTESIAN_POINT('',(50.4902099491237,-15.,104.000005722046));
#5661=CARTESIAN_POINT('',(50.4902099491237,-14.2000010917973,104.799999861885));
#5662=CARTESIAN_POINT('',(50.4902099491237,-13.9999997615814,105.));
#5663=CARTESIAN_POINT('',(50.4902099491237,-16.,104.799999861885));
#5664=CARTESIAN_POINT('Origin',(4.99999870072585,-16.,105.999999909568));
#5665=CARTESIAN_POINT('',(4.99999750863295,-8.,105.999999909568));
#5666=CARTESIAN_POINT('',(4.99999750863295,-8.,105.999999909568));
#5667=CARTESIAN_POINT('',(4.9999981046794,-9.,105.999999909568));
#5668=CARTESIAN_POINT('',(4.99999750863295,-16.,105.999999909568));
#5669=CARTESIAN_POINT('',(4.99999870072585,-16.,105.999999909568));
#5670=CARTESIAN_POINT('',(4.99999870072585,-16.,105.999999909568));
#5671=CARTESIAN_POINT('',(-2.49136704573705E-6,-16.,105.999999909568));
#5672=CARTESIAN_POINT('Origin',(9.9999995652367,-13.2,103.499999046326));
#5673=CARTESIAN_POINT('',(8.24999986969346,-13.2,103.499999046326));
#5674=CARTESIAN_POINT('Origin',(9.9999995652367,-13.2,103.499999046326));
#5675=CARTESIAN_POINT('Origin',(9.9999995652367,-16.,103.499999046326));
#5676=CARTESIAN_POINT('',(8.24999986969346,-8.,103.499999046326));
#5677=CARTESIAN_POINT('',(8.24999986969346,-16.,103.499999046326));
#5678=CARTESIAN_POINT('Origin',(9.9999995652367,-8.,103.499999046326));
#5679=CARTESIAN_POINT('Origin',(75.2228257418789,-16.,100.999999909569));
#5680=CARTESIAN_POINT('',(9.99999750863295,-16.,100.999999909568));
#5681=CARTESIAN_POINT('',(9.99999750863295,-16.,100.999999909568));
#5682=CARTESIAN_POINT('',(9.99999750863295,-9.,100.999999909568));
#5683=CARTESIAN_POINT('',(9.99999750863295,-16.,100.999999909568));
#5684=CARTESIAN_POINT('',(-2.49136704025923E-6,-9.,100.9999995123));
#5685=CARTESIAN_POINT('',(79.9288616965592,-9.00000000000001,100.999999909568));
#5686=CARTESIAN_POINT('',(-2.49136703082233E-6,-8.,100.999999909568));
#5687=CARTESIAN_POINT('',(-2.49136703180205E-6,-16.,100.999999909568));
#5688=CARTESIAN_POINT('',(-2.49136703082233E-6,-8.,100.999999909568));
#5689=CARTESIAN_POINT('Origin',(4.99999750863296,-16.,95.9999999095684));
#5690=CARTESIAN_POINT('',(4.99999750863297,-16.,65.2452060764368));
#5691=CARTESIAN_POINT('',(4.99999750863296,-16.,95.9999999095684));
#5692=CARTESIAN_POINT('',(4.99999750863296,-16.,95.9999999095684));
#5693=CARTESIAN_POINT('',(4.99999750863297,-9.,65.2452060764368));
#5694=CARTESIAN_POINT('',(4.99999750863297,-16.,65.2452060764368));
#5695=CARTESIAN_POINT('',(4.99999750863297,-9.,95.9999999095684));
#5696=CARTESIAN_POINT('',(4.99999750863297,-9.,95.9999999095684));
#5697=CARTESIAN_POINT('',(4.99999750863296,-16.,95.9999999095684));
#5698=CARTESIAN_POINT('Origin',(9.99999750863296,-16.,95.9999999095684));
#5699=CARTESIAN_POINT('Origin',(9.99999750863296,-16.,95.9999999095684));
#5700=CARTESIAN_POINT('Origin',(9.99999750863296,-9.,95.9999999095684));
#5701=CARTESIAN_POINT('Origin',(4.99999750863296,-16.,100.999999909568));
#5702=CARTESIAN_POINT('',(-2.49136704512472E-6,-16.,100.999998717475));
#5703=CARTESIAN_POINT('Origin',(4.99999750863296,-16.,100.999999909568));
#5704=CARTESIAN_POINT('Origin',(4.99999750863297,-8.,100.999999909568));
#5705=CARTESIAN_POINT('',(-2.49136704512472E-6,-16.,100.999998717475));
#5706=CARTESIAN_POINT('Origin',(-2.49136704023105E-6,-16.,61.0401448299175));
#5707=CARTESIAN_POINT('',(-2.49136704023105E-6,-16.,61.0401448299175));
#5708=CARTESIAN_POINT('',(-2.49136703275579E-6,-16.,-3.90512892134431E-6));
#5709=CARTESIAN_POINT('',(-2.4913670393738E-6,-9.,61.0401448299175));
#5710=CARTESIAN_POINT('',(-2.49136703189854E-6,-9.,-3.90512892134431E-6));
#5711=CARTESIAN_POINT('',(-2.49136704023105E-6,-16.,61.0401448299175));
#5712=CARTESIAN_POINT('Origin',(55.4902099491237,-15.,104.000005722046));
#5713=CARTESIAN_POINT('',(60.4902099491237,-16.,104.000005722046));
#5714=CARTESIAN_POINT('',(55.4902099491237,-16.,104.000005722046));
#5715=CARTESIAN_POINT('',(60.4902099491237,-15.,104.000005722046));
#5716=CARTESIAN_POINT('',(60.4902099491237,-15.,104.000005722046));
#5717=CARTESIAN_POINT('',(55.4902099491237,-15.,104.000005722046));
#5718=CARTESIAN_POINT('Origin',(55.4902099491237,-14.2000010917973,104.799999861885));
#5719=CARTESIAN_POINT('',(60.4902099491237,-14.2000010917973,104.799999861885));
#5720=CARTESIAN_POINT('',(60.4902099491237,-13.9999997615814,105.));
#5721=CARTESIAN_POINT('',(57.9902099491237,-14.2000010917973,104.799999861885));
#5722=CARTESIAN_POINT('Origin',(55.4902099491237,-15.,103.000001907349));
#5723=CARTESIAN_POINT('',(60.4902099491237,-14.0786711782186,102.078678577114));
#5724=CARTESIAN_POINT('',(52.9902099491237,-14.0786711782186,102.078678577114));
#5725=CARTESIAN_POINT('',(60.4902099491237,-15.,103.000001907349));
#5726=CARTESIAN_POINT('',(60.4902099491237,-15.,103.000001907349));
#5727=CARTESIAN_POINT('',(55.4902099491237,-15.,103.000001907349));
#5728=CARTESIAN_POINT('Origin',(55.4902099491237,-16.,103.000001907349));
#5729=CARTESIAN_POINT('',(60.4902099491237,-16.,103.000001907349));
#5730=CARTESIAN_POINT('',(60.4902099491237,-17.613291571013,103.000001907349));
#5731=CARTESIAN_POINT('',(55.4902099491237,-16.,103.000001907349));
#5732=CARTESIAN_POINT('Origin',(55.4902099491237,-16.,52.9999980022196));
#5733=CARTESIAN_POINT('',(104.252765939044,-16.,100.878679694998));
#5734=CARTESIAN_POINT('',(20.9321760059474,-16.,17.5580486346965));
#5735=CARTESIAN_POINT('',(102.131450069058,-16.,105.999999909568));
#5736=CARTESIAN_POINT('Origin',(102.131445466495,-16.,102.999999909569));
#5737=CARTESIAN_POINT('',(60.4902099491237,-16.,105.999999909569));
#5738=CARTESIAN_POINT('',(-2.49136704573705E-6,-16.,105.999999909568));
#5739=CARTESIAN_POINT('',(60.4902099491237,-16.,78.7000003970924));
#5740=CARTESIAN_POINT('',(78.0377000859664,-16.,78.199171079613));
#5741=CARTESIAN_POINT('Origin',(19.277688217409,-16.,159.40067439748));
#5742=CARTESIAN_POINT('',(81.3189100147365,-16.,80.6776794482952));
#5743=CARTESIAN_POINT('',(77.8756307483791,-16.,78.0767497112041));
#5744=CARTESIAN_POINT('',(83.2198404193996,-16.,84.6014246036297));
#5745=CARTESIAN_POINT('Origin',(78.2198382097572,-16.,84.6014246036297));
#5746=CARTESIAN_POINT('',(83.2198404193996,-16.,91.2703653861766));
#5747=CARTESIAN_POINT('',(83.2198404193996,-16.,91.2703653861766));
#5748=CARTESIAN_POINT('',(90.0482438923,-16.,88.4419473697429));
#5749=CARTESIAN_POINT('Origin',(87.21982630964,-16.,91.2703640823622));
#5750=CARTESIAN_POINT('',(6.72763826472058,-16.,5.1213161121643));
#5751=CARTESIAN_POINT('',(60.4902099491237,-16.,100.999999909569));
#5752=CARTESIAN_POINT('',(60.4902099491237,-16.,77.5393382896666));
#5753=CARTESIAN_POINT('',(75.2228257418789,-16.,100.999999909569));
#5754=CARTESIAN_POINT('',(9.99999750863295,-16.,100.999999909568));
#5755=CARTESIAN_POINT('',(78.2228256672992,-16.,97.9993309712914));
#5756=CARTESIAN_POINT('Origin',(75.2228257418789,-16.,97.9999999095685));
#5757=CARTESIAN_POINT('',(78.2198380979424,-16.,84.601424987681));
#5758=CARTESIAN_POINT('',(78.2198382097572,-16.,84.6014246036297));
#5759=CARTESIAN_POINT('Origin',(19.277688217409,-16.,159.40067439748));
#5760=CARTESIAN_POINT('Origin',(50.4902099491237,-16.,102.078678577114));
#5761=CARTESIAN_POINT('',(60.4902099491237,-8.00000000000001,102.078678577114));
#5762=CARTESIAN_POINT('',(51.5279657183439,-8.00000000000001,102.078678577114));
#5763=CARTESIAN_POINT('',(60.4902099491237,-16.,102.078678577114));
#5764=CARTESIAN_POINT('Origin',(52.5657214875641,-8.00000000000001,103.499999909568));
#5765=CARTESIAN_POINT('',(60.4902099491237,-8.00000000000001,104.799999861885));
#5766=CARTESIAN_POINT('',(56.5279657183439,-8.00000000000001,104.799999861885));
#5767=CARTESIAN_POINT('',(60.4902099491237,-8.00000000000001,105.999999909569));
#5768=CARTESIAN_POINT('',(60.4902099491237,-8.00000000000001,104.749999909569));
#5769=CARTESIAN_POINT('',(102.131445466495,-8.00000000000001,105.999999909569));
#5770=CARTESIAN_POINT('',(4.99999750863295,-8.,105.999999909568));
#5771=CARTESIAN_POINT('',(104.367513443995,-8.00000000000001,100.999999909568));
#5772=CARTESIAN_POINT('Origin',(102.131445466495,-8.00000000000001,102.999999909569));
#5773=CARTESIAN_POINT('',(60.4902099491237,-8.00000000000001,100.999999909569));
#5774=CARTESIAN_POINT('',(-2.49136703082233E-6,-8.,100.999999909568));
#5775=CARTESIAN_POINT('',(60.4902099491237,-8.00000000000001,102.789339243341));
#5776=CARTESIAN_POINT('Origin',(104.252765939044,-16.,100.878679694998));
#5777=CARTESIAN_POINT('',(104.252765939044,-9.00000000000001,100.878679694998));
#5778=CARTESIAN_POINT('',(20.9321760059474,-9.,17.5580486346965));
#5779=CARTESIAN_POINT('',(104.252765939044,-16.,100.878679694998));
#5780=CARTESIAN_POINT('Origin',(19.277688217409,-16.,159.40067439748));
#5781=CARTESIAN_POINT('',(78.0377000859664,-9.00000000000001,78.199171079613));
#5782=CARTESIAN_POINT('Origin',(19.277688217409,-9.,159.40067439748));
#5783=CARTESIAN_POINT('',(78.0377000859664,-16.,78.199171079613));
#5784=CARTESIAN_POINT('Origin',(55.4902099491237,-9.00000000000001,52.9999980022196));
#5785=CARTESIAN_POINT('',(90.0482438923,-9.00000000000001,88.4419473697429));
#5786=CARTESIAN_POINT('',(6.72763826472058,-9.,5.1213161121643));
#5787=CARTESIAN_POINT('',(83.2198404193996,-9.00000000000001,91.2703653861766));
#5788=CARTESIAN_POINT('Origin',(87.21982630964,-9.00000000000001,91.2703640823622));
#5789=CARTESIAN_POINT('',(83.2198404193996,-9.00000000000001,84.6014246036297));
#5790=CARTESIAN_POINT('',(83.2198404193996,-9.00000000000001,91.2703653861766));
#5791=CARTESIAN_POINT('',(81.3189100147365,-9.00000000000001,80.6776794482952));
#5792=CARTESIAN_POINT('Origin',(78.2198382097572,-9.00000000000001,84.6014246036297));
#5793=CARTESIAN_POINT('',(77.8756307483791,-9.00000000000001,78.0767497112041));
#5794=CARTESIAN_POINT('',(78.2198380979424,-9.00000000000001,84.601424987681));
#5795=CARTESIAN_POINT('Origin',(19.277688217409,-9.,159.40067439748));
#5796=CARTESIAN_POINT('',(78.2228256672992,-9.00000000000001,97.9993309712914));
#5797=CARTESIAN_POINT('',(78.2198382097572,-9.00000000000001,84.6014246036297));
#5798=CARTESIAN_POINT('',(75.2228257418789,-9.00000000000001,100.999999909569));
#5799=CARTESIAN_POINT('Origin',(75.2228257418789,-9.00000000000001,97.9999999095685));
#5800=CARTESIAN_POINT('',(104.367513443995,-9.00000000000001,100.999999909568));
#5801=CARTESIAN_POINT('',(79.9288616965592,-9.00000000000001,100.999999909568));
#5802=CARTESIAN_POINT('Origin',(102.131445466495,-9.00000000000001,102.999999909569));
#5803=CARTESIAN_POINT('Origin',(60.4902099491237,-16.,102.078678577114));
#5804=CARTESIAN_POINT('',(60.4902099491237,-16.,100.999999909569));
#5805=CARTESIAN_POINT('Origin',(60.4902099491237,-16.,104.799999861885));
#5806=CARTESIAN_POINT('',(60.4902099491237,-16.,104.799999861885));
#5807=CARTESIAN_POINT('Origin',(60.4902099491237,-16.,105.999999909569));
#5808=CARTESIAN_POINT('',(60.4902099491237,-16.,105.999999909568));
#5809=CARTESIAN_POINT('Origin',(75.2228257418789,-16.,100.999999909569));
#5810=CARTESIAN_POINT('',(104.367513443995,-16.,100.999999909568));
#5811=CARTESIAN_POINT('',(75.2228257418789,-16.,100.999999909569));
#5812=CARTESIAN_POINT('Origin',(75.2228257418789,-16.,97.9999999095685));
#5813=CARTESIAN_POINT('',(78.2228256672992,-16.,97.9993309712914));
#5814=CARTESIAN_POINT('Origin',(78.2198382097572,-16.,84.6014246036297));
#5815=CARTESIAN_POINT('',(78.2198382097572,-16.,84.6014246036297));
#5816=CARTESIAN_POINT('Origin',(19.277688217409,-16.,159.40067439748));
#5817=CARTESIAN_POINT('Origin',(81.3189100147365,-16.,80.6776794482952));
#5818=CARTESIAN_POINT('',(81.3189100147365,-16.,80.6776794482952));
#5819=CARTESIAN_POINT('Origin',(78.2198382097572,-16.,84.6014246036297));
#5820=CARTESIAN_POINT('',(83.2198404193996,-16.,84.6014246036297));
#5821=CARTESIAN_POINT('Origin',(83.2198404193996,-16.,91.2703653861766));
#5822=CARTESIAN_POINT('',(83.2198404193996,-16.,91.2703653861766));
#5823=CARTESIAN_POINT('Origin',(87.21982630964,-16.,91.2703640823622));
#5824=CARTESIAN_POINT('',(90.0482438923,-16.,88.4419473697429));
#5825=CARTESIAN_POINT('Origin',(4.99999870072585,-16.,105.999999909568));
#5826=CARTESIAN_POINT('',(102.131447767777,-9.00000000000001,105.999999909569));
#5827=CARTESIAN_POINT('',(102.131450069058,-16.,105.999999909568));
#5828=CARTESIAN_POINT('',(102.131445466495,-16.,105.999999909569));
#5829=CARTESIAN_POINT('Origin',(102.131445466495,-16.,102.999999909569));
#5830=CARTESIAN_POINT('Origin',(6.72763826472058,-16.,5.1213161121643));
#5895=UNCERTAINTY_MEASURE_WITH_UNIT(LENGTH_MEASURE(0.01),#5913,
'DISTANCE_ACCURACY_VALUE',
'Maximum model space distance between geometric entities at asserted c
onnectivities');
#5902=UNCERTAINTY_MEASURE_WITH_UNIT(LENGTH_MEASURE(0.01),#5913,
'DISTANCE_ACCURACY_VALUE',
'Maximum model space distance between geometric entities at asserted c
onnectivities');
#5905=(
GEOMETRIC_REPRESENTATION_CONTEXT(3)
GLOBAL_UNCERTAINTY_ASSIGNED_CONTEXT((#5895))
GLOBAL_UNIT_ASSIGNED_CONTEXT((#5913,#5915,#5916))
REPRESENTATION_CONTEXT('','3D')
);
#5912=(
GEOMETRIC_REPRESENTATION_CONTEXT(3)
GLOBAL_UNCERTAINTY_ASSIGNED_CONTEXT((#5902))
GLOBAL_UNIT_ASSIGNED_CONTEXT((#5913,#5915,#5916))
REPRESENTATION_CONTEXT('','3D')
);
#5913=(
LENGTH_UNIT()
NAMED_UNIT(*)
SI_UNIT(.MILLI.,.METRE.)
);
#5915=(
NAMED_UNIT(*)
PLANE_ANGLE_UNIT()
SI_UNIT($,.RADIAN.)
);
#5916=(
NAMED_UNIT(*)
SI_UNIT($,.STERADIAN.)
SOLID_ANGLE_UNIT()
);
#5919=SHAPE_DEFINITION_REPRESENTATION(#5928,#5945);
#5928=PRODUCT_DEFINITION_SHAPE('',$,#5955);
#5945=SHAPE_REPRESENTATION('',(#3704),#5905);
#5952=PRODUCT_DEFINITION_CONTEXT('part definition',#5981,'design');
#5955=PRODUCT_DEFINITION('Right_Part','Right_Part',#5964,#5952);
#5964=PRODUCT_DEFINITION_FORMATION('',$,#5985);
#5981=APPLICATION_CONTEXT(
'Core Data for Automotive Mechanical Design Process');
#5982=PRODUCT_CONTEXT('part definition',#5981,'mechanical');
#5985=PRODUCT('Right_Part','Right_Part',$,(#5982));
#5993=PRESENTATION_STYLE_ASSIGNMENT((#5996));
#5996=SURFACE_STYLE_USAGE(.BOTH.,#5999);
#5999=SURFACE_SIDE_STYLE('',(#6002));
#6002=SURFACE_STYLE_FILL_AREA(#6005);
#6005=FILL_AREA_STYLE('Opaque(179,179,179)',(#6008));
#6008=FILL_AREA_STYLE_COLOUR('Opaque(179,179,179)',#6011);
#6011=COLOUR_RGB('Opaque(179,179,179)', 0.09019608, 0.27058824, 0.51372549);
ENDSEC;
END-ISO-10303-21;
